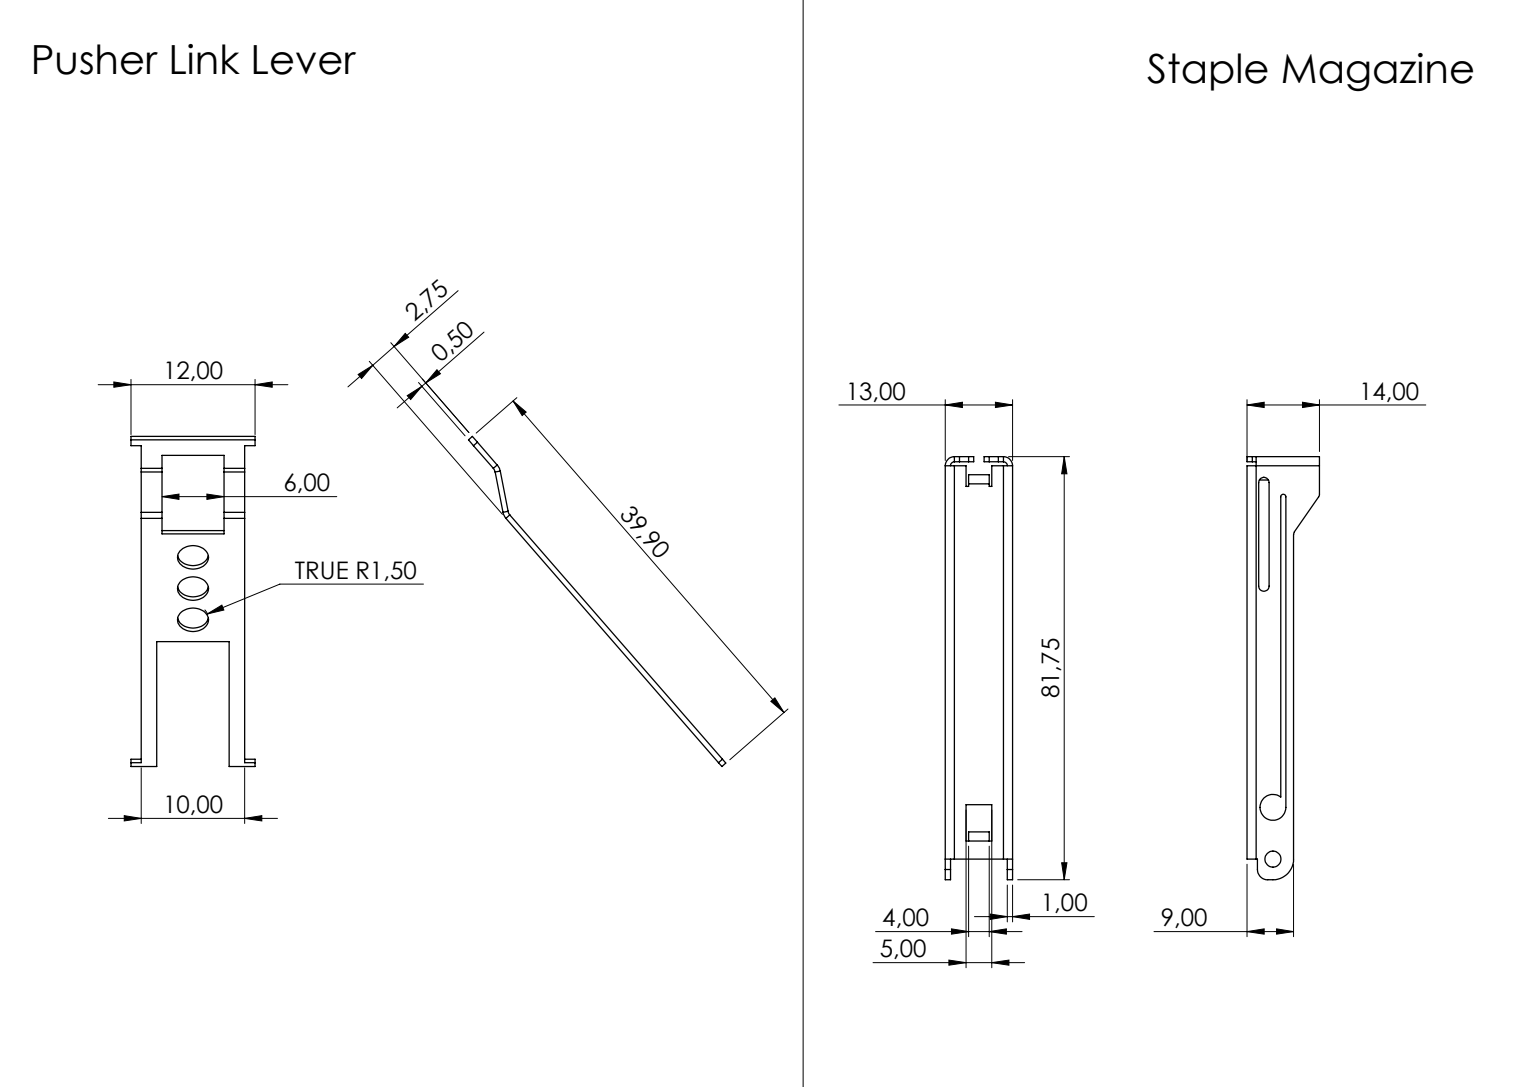
ISO-10303-21;
HEADER;
FILE_DESCRIPTION (('STEP AP214'),
    '1' );
FILE_NAME ('Pusher Link Lever.step',
    '2026-10-06T10:23:46',
    ( '' ),
    ( '' ),
    'SwSTEP 2.0',
    'SolidWorks 2020',
    '' );
FILE_SCHEMA (( 'AUTOMOTIVE_DESIGN' ));
ENDSEC;

DATA;
#10=VECTOR ( 'NONE', #20731, 1000.000000000000000 ) ;
#51=VECTOR ( 'NONE', #12391, 1000.000000000000227 ) ;
#60=CARTESIAN_POINT ( 'NONE',  ( 41.31606138205700063, 9.119667998728431257, 66.98393923633439329 ) ) ;
#67=CARTESIAN_POINT ( 'NONE',  ( 33.31606138205700773, -20.55619265724211076, 44.11584019928223910 ) ) ;
#85=CARTESIAN_POINT ( 'NONE',  ( 33.31606138205700773, -20.55619265724211076, 44.11584019928223910 ) ) ;
#88=CARTESIAN_POINT ( 'NONE',  ( 33.31606138205700773, 7.043113989679085307, 66.83274420321491505 ) ) ;
#111=EDGE_CURVE ( 'NONE', #24693, #6631, #6848, .T. ) ;
#114=EDGE_CURVE ( 'NONE', #23891, #14933, #22516, .T. ) ;
#137=SURFACE_STYLE_USAGE ( .BOTH. , #13306 ) ;
#149=DIRECTION ( 'NONE',  ( 0.000000000000000000, -0.7540134720837687876, -0.6568589528324780824 ) ) ;
#159=CARTESIAN_POINT ( 'NONE',  ( 41.31606138205700063, 7.187001342539796944, 66.09667597968754649 ) ) ;
#171=CARTESIAN_POINT ( 'NONE',  ( 43.31606138205700063, 3.536347952325769040, 64.10938348997790115 ) ) ;
#176=DIRECTION ( 'NONE',  ( 0.000000000000000000, 0.9814242980364923374, 0.1918498038142812112 ) ) ;
#215=LINE ( 'NONE', #15932, #731 ) ;
#239=ORIENTED_EDGE ( 'NONE', *, *, #12746, .F. ) ;
#276=CARTESIAN_POINT ( 'NONE',  ( 33.31606138205700773, -21.26162886970023536, 44.16441745890789150 ) ) ;
#333=EDGE_CURVE ( 'NONE', #14933, #7242, #7489, .T. ) ;
#339=EDGE_LOOP ( 'NONE', ( #14146, #23745, #1697, #21573 ) ) ;
#370=AXIS2_PLACEMENT_3D ( 'NONE', #22891, #22513, #18525 ) ;
#381=LINE ( 'NONE', #10079, #6023 ) ;
#388=ADVANCED_FACE ( 'NONE', ( #12254 ), #16230, .F. ) ;
#398=ORIENTED_EDGE ( 'NONE', *, *, #4868, .T. ) ;
#411=VECTOR ( 'NONE', #3457, 1000.000000000000227 ) ;
#416=DIRECTION ( 'NONE',  ( -1.000000000000000000, 0.000000000000000000, 0.000000000000000000 ) ) ;
#423=VECTOR ( 'NONE', #2307, 1000.000000000000000 ) ;
#432=EDGE_LOOP ( 'NONE', ( #18216, #5933, #5741, #16372 ) ) ;
#465=DIRECTION ( 'NONE',  ( 0.000000000000000000, -0.1918498038142812112, 0.9814242980364923374 ) ) ;
#484=DIRECTION ( 'NONE',  ( -1.000000000000000000, 0.000000000000000000, 0.000000000000000000 ) ) ;
#512=VECTOR ( 'NONE', #1905, 1000.000000000000227 ) ;
#522=DIRECTION ( 'NONE',  ( -1.000000000000000000, 0.000000000000000000, 0.000000000000000000 ) ) ;
#532=FACE_BOUND ( 'NONE', #6040, .T. ) ;
#572=CARTESIAN_POINT ( 'NONE',  ( 32.31606138205700063, -20.55619265724211076, 44.11584019928223910 ) ) ;
#583=EDGE_CURVE ( 'NONE', #22400, #7712, #22663, .T. ) ;
#586=DIRECTION ( 'NONE',  ( 0.000000000000000000, -0.7540134720837717852, -0.6568589528324746407 ) ) ;
#606=CARTESIAN_POINT ( 'NONE',  ( 41.31606138205700063, 7.864187680719676443, 65.89022736311019912 ) ) ;
#609=FACE_OUTER_BOUND ( 'NONE', #22404, .T. ) ;
#626=LINE ( 'NONE', #2187, #423 ) ;
#634=LINE ( 'NONE', #22037, #2547 ) ;
#649=EDGE_CURVE ( 'NONE', #18044, #10390, #12216, .T. ) ;
#676=DIRECTION ( 'NONE',  ( 1.000000000000000000, 0.000000000000000000, 0.000000000000000000 ) ) ;
#684=LINE ( 'NONE', #8319, #13350 ) ;
#692=EDGE_LOOP ( 'NONE', ( #13673, #1108, #11272, #13353 ) ) ;
#698=DIRECTION ( 'NONE',  ( 0.000000000000000000, -0.6568589528324746407, 0.7540134720837716742 ) ) ;
#708=PLANE ( 'NONE',  #13919 ) ;
#718=EDGE_LOOP ( 'NONE', ( #8864, #2817, #9327, #12481 ) ) ;
#731=VECTOR ( 'NONE', #465, 1000.000000000000227 ) ;
#746=ORIENTED_EDGE ( 'NONE', *, *, #3453, .F. ) ;
#758=EDGE_CURVE ( 'NONE', #12000, #4126, #215, .T. ) ;
#773=ORIENTED_EDGE ( 'NONE', *, *, #17559, .F. ) ;
#802=EDGE_CURVE ( 'NONE', #973, #13467, #6103, .T. ) ;
#815=ORIENTED_EDGE ( 'NONE', *, *, #8639, .F. ) ;
#866=ADVANCED_FACE ( 'NONE', ( #9118 ), #22748, .T. ) ;
#893=DIRECTION ( 'NONE',  ( -1.000000000000000000, 0.000000000000000000, 0.000000000000000000 ) ) ;
#909=CARTESIAN_POINT ( 'NONE',  ( 39.81606138205700063, -1.383222575549920119, 62.14461230196212682 ) ) ;
#963=CARTESIAN_POINT ( 'NONE',  ( 35.31606138205700773, 3.043703737701412226, 64.67489359404071081 ) ) ;
#970=CARTESIAN_POINT ( 'NONE',  ( 33.31606138205700773, 3.392460599465057403, 64.84545171350526971 ) ) ;
#973=VERTEX_POINT ( 'NONE', #15403 ) ;
#979=MECHANICAL_DESIGN_GEOMETRIC_PRESENTATION_REPRESENTATION('',(#16209),#14965);
#981=VERTEX_POINT ( 'NONE', #23370 ) ;
#995=FACE_BOUND ( 'NONE', #20971, .T. ) ;
#1028=ORIENTED_EDGE ( 'NONE', *, *, #24774, .T. ) ;
#1039=CARTESIAN_POINT ( 'NONE',  ( 41.31606138205700063, 8.104266321858618838, 55.82104096753806033 ) ) ;
#1091=CARTESIAN_POINT ( 'NONE',  ( 44.31606138205700063, 10.06218483883314718, 67.80501292737497465 ) ) ;
#1093=FACE_OUTER_BOUND ( 'NONE', #22758, .T. ) ;
#1095=DIRECTION ( 'NONE',  ( 0.000000000000000000, 0.7540134720837716742, 0.6568589528324746407 ) ) ;
#1108=ORIENTED_EDGE ( 'NONE', *, *, #23862, .T. ) ;
#1117=ADVANCED_FACE ( 'NONE', ( #22102 ), #16173, .F. ) ;
#1123=PLANE ( 'NONE',  #20476 ) ;
#1127=DIRECTION ( 'NONE',  ( 0.000000000000000000, 0.7540134720837716742, 0.6568589528324746407 ) ) ;
#1149=DIRECTION ( 'NONE',  ( 0.000000000000000000, 0.7540134720837716742, 0.6568589528324746407 ) ) ;
#1181=CIRCLE ( 'NONE', #15586, 1.500000000000001332 ) ;
#1206=FACE_OUTER_BOUND ( 'NONE', #18017, .T. ) ;
#1208=ORIENTED_EDGE ( 'NONE', *, *, #18160, .F. ) ;
#1241=ADVANCED_BREP_SHAPE_REPRESENTATION ( '', ( #17413, #2000 ), #7588 ) ;
#1245=ORIENTED_EDGE ( 'NONE', *, *, #19719, .F. ) ;
#1253=VECTOR ( 'NONE', #12245, 1000.000000000000227 ) ;
#1256=CARTESIAN_POINT ( 'NONE',  ( 33.31606138205700773, 10.62769494289597993, 68.29765714199933768 ) ) ;
#1260=LINE ( 'NONE', #24820, #4453 ) ;
#1265=CARTESIAN_POINT ( 'NONE',  ( 41.81606138205700063, -14.36460986495925241, 36.24727600202827915 ) ) ;
#1296=VERTEX_POINT ( 'NONE', #10772 ) ;
#1345=LINE ( 'NONE', #22733, #4452 ) ;
#1354=ORIENTED_EDGE ( 'NONE', *, *, #20276, .F. ) ;
#1382=ORIENTED_EDGE ( 'NONE', *, *, #10274, .T. ) ;
#1383=FACE_OUTER_BOUND ( 'NONE', #17604, .T. ) ;
#1395=EDGE_CURVE ( 'NONE', #20256, #6631, #1345, .T. ) ;
#1401=AXIS2_PLACEMENT_3D ( 'NONE', #3846, #7337, #9406 ) ;
#1404=ORIENTED_EDGE ( 'NONE', *, *, #22708, .F. ) ;
#1426=CARTESIAN_POINT ( 'NONE',  ( 43.31606138205700063, 7.535758204303438568, 66.26723409915207696 ) ) ;
#1453=ADVANCED_FACE ( 'NONE', ( #19133 ), #17457, .T. ) ;
#1471=FACE_OUTER_BOUND ( 'NONE', #24405, .T. ) ;
#1479=CARTESIAN_POINT ( 'NONE',  ( 33.31606138205700773, 7.282926244446933595, 65.60596383066929604 ) ) ;
#1497=CARTESIAN_POINT ( 'NONE',  ( 33.31606138205700773, -20.93319939328399926, 43.78741072286599945 ) ) ;
#1504=ADVANCED_FACE ( 'NONE', ( #3782 ), #23485, .F. ) ;
#1518=CARTESIAN_POINT ( 'NONE',  ( 33.31606138205700773, 7.535758204303438568, 66.26723409915207696 ) ) ;
#1524=CARTESIAN_POINT ( 'NONE',  ( 34.81606138205700773, -20.93319939328399926, 43.78741072286599945 ) ) ;
#1549=FACE_OUTER_BOUND ( 'NONE', #339, .T. ) ;
#1554=CARTESIAN_POINT ( 'NONE',  ( 33.31606138205700773, 7.864187680719676443, 65.89022736311019912 ) ) ;
#1555=EDGE_CURVE ( 'NONE', #18393, #21009, #3531, .T. ) ;
#1556=CARTESIAN_POINT ( 'NONE',  ( 35.31606138205700773, 7.283211578144648257, 66.04722806671131252 ) ) ;
#1567=CARTESIAN_POINT ( 'NONE',  ( 33.31606138205700773, 3.536347952325769040, 64.10938348997790115 ) ) ;
#1611=ORIENTED_EDGE ( 'NONE', *, *, #17429, .F. ) ;
#1641=FACE_OUTER_BOUND ( 'NONE', #23272, .T. ) ;
#1655=ORIENTED_EDGE ( 'NONE', *, *, #17523, .T. ) ;
#1664=EDGE_LOOP ( 'NONE', ( #7698, #19659, #15384, #19509 ) ) ;
#1697=ORIENTED_EDGE ( 'NONE', *, *, #18160, .T. ) ;
#1709=CARTESIAN_POINT ( 'NONE',  ( 38.31606138205700063, -4.399276463885007260, 59.51717649063222382 ) ) ;
#1710=VECTOR ( 'NONE', #11846, 1000.000000000000227 ) ;
#1719=ORIENTED_EDGE ( 'NONE', *, *, #7493, .T. ) ;
#1756=EDGE_CURVE ( 'NONE', #3936, #14994, #21690, .T. ) ;
#1793=VERTEX_POINT ( 'NONE', #4682 ) ;
#1808=VECTOR ( 'NONE', #12372, 1000.000000000000227 ) ;
#1812=CARTESIAN_POINT ( 'NONE',  ( 35.31606138205700773, 7.043113989679085307, 66.83274420321491505 ) ) ;
#1827=DIRECTION ( 'NONE',  ( 0.000000000000000000, 0.7540134720837716742, 0.6568589528324746407 ) ) ;
#1859=EDGE_CURVE ( 'NONE', #16267, #9779, #14977, .T. ) ;
#1867=ORIENTED_EDGE ( 'NONE', *, *, #17709, .T. ) ;
#1870=LINE ( 'NONE', #17869, #4225 ) ;
#1871=ORIENTED_EDGE ( 'NONE', *, *, #114, .T. ) ;
#1896=ORIENTED_EDGE ( 'NONE', *, *, #14372, .F. ) ;
#1905=DIRECTION ( 'NONE',  ( 5.421010862427517856E-17, -0.7540134720837717852, -0.6568589528324746407 ) ) ;
#1909=( LENGTH_UNIT ( ) NAMED_UNIT ( * ) SI_UNIT ( .MILLI., .METRE. ) );
#1912=DIRECTION ( 'NONE',  ( -1.000000000000000000, 0.000000000000000000, 0.000000000000000000 ) ) ;
#1916=DIRECTION ( 'NONE',  ( 0.000000000000000000, 0.7540134720837725624, 0.6568589528324736415 ) ) ;
#1919=ORIENTED_EDGE ( 'NONE', *, *, #12872, .F. ) ;
#1947=DIRECTION ( 'NONE',  ( 0.000000000000000000, 0.6568589528324746407, -0.7540134720837716742 ) ) ;
#1962=CARTESIAN_POINT ( 'NONE',  ( 35.31606138205700773, 8.104266321858618838, 55.82104096753806033 ) ) ;
#1979=EDGE_CURVE ( 'NONE', #2339, #23360, #5441, .T. ) ;
#1997=VERTEX_POINT ( 'NONE', #13310 ) ;
#2000=AXIS2_PLACEMENT_3D ( 'NONE', #9286, #12766, #22537 ) ;
#2004=DIRECTION ( 'NONE',  ( 1.000000000000000000, 0.000000000000000000, 0.000000000000000000 ) ) ;
#2032=VECTOR ( 'NONE', #13072, 1000.000000000000227 ) ;
#2046=AXIS2_PLACEMENT_3D ( 'NONE', #24848, #6964, #1149 ) ;
#2055=VECTOR ( 'NONE', #19199, 1000.000000000000227 ) ;
#2081=EDGE_CURVE ( 'NONE', #22220, #12980, #20869, .T. ) ;
#2084=EDGE_LOOP ( 'NONE', ( #8923, #5906, #22734, #17854 ) ) ;
#2088=PLANE ( 'NONE',  #25150 ) ;
#2111=EDGE_LOOP ( 'NONE', ( #21458, #24071, #20598, #8543 ) ) ;
#2116=ORIENTED_EDGE ( 'NONE', *, *, #7384, .F. ) ;
#2160=VECTOR ( 'NONE', #13117, 1000.000000000000000 ) ;
#2170=SURFACE_STYLE_USAGE ( .BOTH. , #11599 ) ;
#2178=VECTOR ( 'NONE', #12286, 1000.000000000000227 ) ;
#2187=CARTESIAN_POINT ( 'NONE',  ( 33.31606138205700773, 3.043703737701412226, 64.67489359404071081 ) ) ;
#2190=VERTEX_POINT ( 'NONE', #25289 ) ;
#2196=CARTESIAN_POINT ( 'NONE',  ( 38.31606138205700063, -1.054793099133682244, 61.76760556592023477 ) ) ;
#2222=ORIENTED_EDGE ( 'NONE', *, *, #20103, .F. ) ;
#2226=DIRECTION ( 'NONE',  ( 0.000000000000000000, 0.7540134720837717852, 0.6568589528324746407 ) ) ;
#2242=DIRECTION ( 'NONE',  ( 0.000000000000000000, -0.6568589528324746407, 0.7540134720837717852 ) ) ;
#2264=ORIENTED_EDGE ( 'NONE', *, *, #12872, .T. ) ;
#2265=CARTESIAN_POINT ( 'NONE',  ( 33.31606138205700773, 3.099306811489555891, 65.29760936252343129 ) ) ;
#2289=ADVANCED_FACE ( 'NONE', ( #15510 ), #13347, .T. ) ;
#2298=EDGE_LOOP ( 'NONE', ( #9215, #19456, #10247, #6097 ) ) ;
#2307=DIRECTION ( 'NONE',  ( 1.000000000000000000, 0.000000000000000000, 0.000000000000000000 ) ) ;
#2311=CARTESIAN_POINT ( 'NONE',  ( 43.31606138205700063, 2.715274261285174351, 65.05190033008260286 ) ) ;
#2339=VERTEX_POINT ( 'NONE', #4565 ) ;
#2366=CARTESIAN_POINT ( 'NONE',  ( 43.31606138205700063, 7.043113989679085307, 66.83274420321491505 ) ) ;
#2398=LINE ( 'NONE', #19807, #6565 ) ;
#2403=CARTESIAN_POINT ( 'NONE',  ( 44.31606138205700063, 10.62769494289597993, 68.29765714199933768 ) ) ;
#2409=DIRECTION ( 'NONE',  ( 0.000000000000000000, -0.6568589528324746407, 0.7540134720837717852 ) ) ;
#2420=CIRCLE ( 'NONE', #20143, 1.500000000000001332 ) ;
#2426=EDGE_LOOP ( 'NONE', ( #3479, #7297, #23375, #11174 ) ) ;
#2430=ORIENTED_EDGE ( 'NONE', *, *, #20190, .F. ) ;
#2440=CARTESIAN_POINT ( 'NONE',  ( 33.31606138205700773, -20.93319939328399926, 43.78741072286599945 ) ) ;
#2457=EDGE_CURVE ( 'NONE', #8692, #22403, #21950, .T. ) ;
#2488=ADVANCED_FACE ( 'NONE', ( #24748 ), #9075, .T. ) ;
#2511=ORIENTED_EDGE ( 'NONE', *, *, #19188, .T. ) ;
#2513=EDGE_LOOP ( 'NONE', ( #25331, #17268, #5891, #10881 ) ) ;
#2534=LINE ( 'NONE', #606, #24325 ) ;
#2547=VECTOR ( 'NONE', #4398, 1000.000000000000227 ) ;
#2554=CARTESIAN_POINT ( 'NONE',  ( 33.31606138205700773, 10.06218483883314718, 67.80501292737497465 ) ) ;
#2563=DIRECTION ( 'NONE',  ( 1.000000000000000000, 0.000000000000000000, 0.000000000000000000 ) ) ;
#2569=CARTESIAN_POINT ( 'NONE',  ( 41.31606138205700063, 7.282926244446937147, 65.60596383066929604 ) ) ;
#2572=VECTOR ( 'NONE', #586, 1000.000000000000227 ) ;
#2573=AXIS2_PLACEMENT_3D ( 'NONE', #16977, #2914, #7188 ) ;
#2591=PLANE ( 'NONE',  #21386 ) ;
#2592=CARTESIAN_POINT ( 'NONE',  ( 33.31606138205700773, 9.733755362416909307, 68.18201966341686671 ) ) ;
#2616=DIRECTION ( 'NONE',  ( 1.000000000000000000, 0.000000000000000000, 0.000000000000000000 ) ) ;
#2633=DIRECTION ( 'NONE',  ( 0.000000000000000000, -0.6568589528324746407, 0.7540134720837717852 ) ) ;
#2637=CARTESIAN_POINT ( 'NONE',  ( 34.81606138205700773, -14.36460986495925241, 36.24727600202827915 ) ) ;
#2639=DIRECTION ( 'NONE',  ( 1.000000000000000000, 0.000000000000000000, 0.000000000000000000 ) ) ;
#2667=ADVANCED_FACE ( 'NONE', ( #7502 ), #7762, .F. ) ;
#2677=CYLINDRICAL_SURFACE ( 'NONE', #16859, 1.500000000000001332 ) ;
#2679=ORIENTED_EDGE ( 'NONE', *, *, #22395, .T. ) ;
#2747=ORIENTED_EDGE ( 'NONE', *, *, #17523, .F. ) ;
#2785=EDGE_CURVE ( 'NONE', #14994, #22403, #21662, .T. ) ;
#2795=EDGE_CURVE ( 'NONE', #14933, #23891, #24552, .T. ) ;
#2797=EDGE_CURVE ( 'NONE', #24510, #23124, #12269, .T. ) ;
#2807=EDGE_LOOP ( 'NONE', ( #24648, #21947 ) ) ;
#2817=ORIENTED_EDGE ( 'NONE', *, *, #11715, .T. ) ;
#2825=LINE ( 'NONE', #18691, #10863 ) ;
#2892=PLANE ( 'NONE',  #9807 ) ;
#2897=LINE ( 'NONE', #8596, #20978 ) ;
#2914=DIRECTION ( 'NONE',  ( 1.000000000000000000, 0.000000000000000000, 0.000000000000000000 ) ) ;
#2937=DIRECTION ( 'NONE',  ( 0.000000000000000000, 0.7540134720837717852, 0.6568589528324745297 ) ) ;
#2965=ADVANCED_FACE ( 'NONE', ( #6079 ), #23962, .T. ) ;
#3009=VECTOR ( 'NONE', #8392, 1000.000000000000000 ) ;
#3043=VERTEX_POINT ( 'NONE', #14563 ) ;
#3061=ADVANCED_FACE ( 'NONE', ( #3088 ), #14685, .T. ) ;
#3064=CARTESIAN_POINT ( 'NONE',  ( 41.31606138205700063, 7.187001342539796944, 66.09667597968754649 ) ) ;
#3065=DIRECTION ( 'NONE',  ( 1.000000000000000000, 0.000000000000000000, 0.000000000000000000 ) ) ;
#3088=FACE_OUTER_BOUND ( 'NONE', #13458, .T. ) ;
#3150=CARTESIAN_POINT ( 'NONE',  ( 35.31606138205700773, 9.119667998728431257, 66.98393923633439329 ) ) ;
#3164=ORIENTED_EDGE ( 'NONE', *, *, #14530, .F. ) ;
#3174=ORIENTED_EDGE ( 'NONE', *, *, #22025, .F. ) ;
#3200=VECTOR ( 'NONE', #4429, 1000.000000000000227 ) ;
#3214=CARTESIAN_POINT ( 'NONE',  ( 35.31606138205700773, 7.282926244446937147, 65.60596383066929604 ) ) ;
#3233=PLANE ( 'NONE',  #23657 ) ;
#3245=DIRECTION ( 'NONE',  ( 0.000000000000000000, -0.7540134720837725624, -0.6568589528324736415 ) ) ;
#3291=CARTESIAN_POINT ( 'NONE',  ( 39.81606138205700063, -4.399276463885007260, 59.51717649063222382 ) ) ;
#3292=VECTOR ( 'NONE', #676, 1000.000000000000000 ) ;
#3304=ORIENTED_EDGE ( 'NONE', *, *, #20261, .T. ) ;
#3307=PLANE ( 'NONE',  #11587 ) ;
#3316=ADVANCED_FACE ( 'NONE', ( #21378 ), #13279, .F. ) ;
#3318=DIRECTION ( 'NONE',  ( 0.000000000000000000, 0.7540134720837716742, 0.6568589528324746407 ) ) ;
#3322=CARTESIAN_POINT ( 'NONE',  ( 38.31606138205700063, -7.415330352220093069, 56.88974067930232081 ) ) ;
#3353=EDGE_CURVE ( 'NONE', #17400, #19611, #1181, .T. ) ;
#3382=PRODUCT_CONTEXT ( 'NONE', #16546, 'mechanical' ) ;
#3389=DIRECTION ( 'NONE',  ( 0.000000000000000000, -0.7540134720837687876, -0.6568589528324780824 ) ) ;
#3403=ORIENTED_EDGE ( 'NONE', *, *, #14691, .F. ) ;
#3420=LINE ( 'NONE', #15017, #22147 ) ;
#3436=VECTOR ( 'NONE', #14093, 1000.000000000000227 ) ;
#3453=EDGE_CURVE ( 'NONE', #21357, #19154, #11862, .T. ) ;
#3454=DIRECTION ( 'NONE',  ( 0.000000000000000000, 0.6568589528324746407, -0.7540134720837717852 ) ) ;
#3457=DIRECTION ( 'NONE',  ( 0.000000000000000000, 0.7540134720837717852, 0.6568589528324746407 ) ) ;
#3479=ORIENTED_EDGE ( 'NONE', *, *, #17709, .F. ) ;
#3496=DIRECTION ( 'NONE',  ( 1.000000000000000000, 0.000000000000000000, 0.000000000000000000 ) ) ;
#3499=PRESENTATION_STYLE_ASSIGNMENT (( #137 ) ) ;
#3502=EDGE_CURVE ( 'NONE', #25135, #22767, #14035, .T. ) ;
#3517=ORIENTED_EDGE ( 'NONE', *, *, #24069, .F. ) ;
#3521=ORIENTED_EDGE ( 'NONE', *, *, #5510, .T. ) ;
#3523=DIRECTION ( 'NONE',  ( 0.000000000000000000, 0.7540134720837716742, 0.6568589528324746407 ) ) ;
#3531=LINE ( 'NONE', #11405, #13900 ) ;
#3564=DIRECTION ( 'NONE',  ( 0.000000000000000000, 0.1918498038142812112, -0.9814242980364923374 ) ) ;
#3586=AXIS2_PLACEMENT_3D ( 'NONE', #14833, #7241, #6984 ) ;
#3627=SHAPE_DEFINITION_REPRESENTATION ( #13836, #18165 ) ;
#3648=AXIS2_PLACEMENT_3D ( 'NONE', #15451, #11350, #17262 ) ;
#3657=DIRECTION ( 'NONE',  ( 0.000000000000000000, 0.6568589528324747517, -0.7540134720837717852 ) ) ;
#3663=ORIENTED_EDGE ( 'NONE', *, *, #11953, .T. ) ;
#3669=ORIENTED_EDGE ( 'NONE', *, *, #11478, .F. ) ;
#3677=CIRCLE ( 'NONE', #370, 0.7500000000000014433 ) ;
#3698=AXIS2_PLACEMENT_3D ( 'NONE', #2196, #17674, #4011 ) ;
#3707=CIRCLE ( 'NONE', #22642, 0.7500000000000014433 ) ;
#3716=CARTESIAN_POINT ( 'NONE',  ( 43.31606138205700063, 7.864187680719676443, 65.89022736311019912 ) ) ;
#3719=EDGE_CURVE ( 'NONE', #17105, #16154, #6279, .T. ) ;
#3721=FILL_AREA_STYLE ('',( #6179 ) ) ;
#3730=EDGE_CURVE ( 'NONE', #24147, #18393, #12212, .T. ) ;
#3782=FACE_OUTER_BOUND ( 'NONE', #23471, .T. ) ;
#3793=CARTESIAN_POINT ( 'NONE',  ( 33.31606138205700773, 7.187001342539796944, 66.09667597968754649 ) ) ;
#3797=CARTESIAN_POINT ( 'NONE',  ( 41.31606138205700063, 3.392460599465057403, 64.84545171350526971 ) ) ;
#3801=CARTESIAN_POINT ( 'NONE',  ( 41.31606138205700063, 7.283211578144648257, 66.04722806671131252 ) ) ;
#3811=PLANE ( 'NONE',  #7511 ) ;
#3844=ORIENTED_EDGE ( 'NONE', *, *, #9003, .F. ) ;
#3846=CARTESIAN_POINT ( 'NONE',  ( 41.31606138205700063, 8.104266321858618838, 55.82104096753806033 ) ) ;
#3850=CARTESIAN_POINT ( 'NONE',  ( 33.31606138205700773, -20.88462213365835041, 44.49284693532412405 ) ) ;
#3907=EDGE_CURVE ( 'NONE', #10892, #20855, #23427, .T. ) ;
#3921=VECTOR ( 'NONE', #4641, 1000.000000000000000 ) ;
#3936=VERTEX_POINT ( 'NONE', #5789 ) ;
#3946=FACE_OUTER_BOUND ( 'NONE', #19029, .T. ) ;
#4011=DIRECTION ( 'NONE',  ( -1.000000000000000000, 0.000000000000000000, 0.000000000000000000 ) ) ;
#4012=CARTESIAN_POINT ( 'NONE',  ( 39.81606138205700063, -1.054793099133682244, 61.76760556592023477 ) ) ;
#4016=CARTESIAN_POINT ( 'NONE',  ( 33.31606138205700773, -21.26162886970023536, 44.16441745890789150 ) ) ;
#4042=CARTESIAN_POINT ( 'NONE',  ( 41.81606138205700063, -14.36460986495925241, 36.24727600202827915 ) ) ;
#4057=CARTESIAN_POINT ( 'NONE',  ( 43.31606138205700063, 3.043703737701412226, 64.67489359404071081 ) ) ;
#4064=DIRECTION ( 'NONE',  ( 0.000000000000000000, 0.6568589528324745297, -0.7540134720837717852 ) ) ;
#4065=ORIENTED_EDGE ( 'NONE', *, *, #24069, .T. ) ;
#4095=CARTESIAN_POINT ( 'NONE',  ( 35.31606138205700773, 3.392460599465057403, 64.84545171350526971 ) ) ;
#4110=AXIS2_PLACEMENT_3D ( 'NONE', #11177, #21088, #7042 ) ;
#4114=EDGE_CURVE ( 'NONE', #6859, #24693, #15194, .T. ) ;
#4119=CIRCLE ( 'NONE', #3698, 1.500000000000001332 ) ;
#4120=DIRECTION ( 'NONE',  ( 0.000000000000000000, 0.6568589528324746407, -0.7540134720837716742 ) ) ;
#4126=VERTEX_POINT ( 'NONE', #19027 ) ;
#4152=DIRECTION ( 'NONE',  ( 0.000000000000000000, -0.6568589528324746407, 0.7540134720837716742 ) ) ;
#4159=DIRECTION ( 'NONE',  ( 0.000000000000000000, 0.7540134720837717852, 0.6568589528324745297 ) ) ;
#4170=ORIENTED_EDGE ( 'NONE', *, *, #10595, .F. ) ;
#4181=CARTESIAN_POINT ( 'NONE',  ( 44.31606138205700063, -20.93319939328399926, 43.78741072286599945 ) ) ;
#4188=LINE ( 'NONE', #4057, #10491 ) ;
#4217=CARTESIAN_POINT ( 'NONE',  ( 39.81606138205700063, -7.415330352220093069, 56.88974067930232081 ) ) ;
#4225=VECTOR ( 'NONE', #11817, 1000.000000000000000 ) ;
#4232=EDGE_CURVE ( 'NONE', #10390, #2339, #4704, .T. ) ;
#4233=EDGE_LOOP ( 'NONE', ( #10281, #1028, #23778, #3174 ) ) ;
#4245=CARTESIAN_POINT ( 'NONE',  ( 41.81606138205700063, -9.197413316359888569, 54.67416070422748220 ) ) ;
#4279=CARTESIAN_POINT ( 'NONE',  ( 33.31606138205700773, 3.099306811489555891, 65.29760936252343129 ) ) ;
#4298=VECTOR ( 'NONE', #6505, 1000.000000000000227 ) ;
#4348=CARTESIAN_POINT ( 'NONE',  ( 33.31606138205700773, -8.868983839943650693, 54.29715396818559725 ) ) ;
#4369=EDGE_CURVE ( 'NONE', #23360, #22220, #7265, .T. ) ;
#4383=VERTEX_POINT ( 'NONE', #10883 ) ;
#4398=DIRECTION ( 'NONE',  ( 0.000000000000000000, -0.7540134720837717852, -0.6568589528324746407 ) ) ;
#4422=ORIENTED_EDGE ( 'NONE', *, *, #14978, .T. ) ;
#4429=DIRECTION ( 'NONE',  ( 0.000000000000000000, -0.6568589528324746407, 0.7540134720837717852 ) ) ;
#4452=VECTOR ( 'NONE', #5098, 1000.000000000000227 ) ;
#4453=VECTOR ( 'NONE', #10201, 1000.000000000000227 ) ;
#4455=ORIENTED_EDGE ( 'NONE', *, *, #19188, .F. ) ;
#4477=DIRECTION ( 'NONE',  ( 0.000000000000000000, 0.7540134720837717852, 0.6568589528324746407 ) ) ;
#4488=ORIENTED_EDGE ( 'NONE', *, *, #10233, .T. ) ;
#4503=ORIENTED_EDGE ( 'NONE', *, *, #333, .F. ) ;
#4515=DIRECTION ( 'NONE',  ( 0.000000000000000000, 0.7540134720837717852, 0.6568589528324747517 ) ) ;
#4522=EDGE_CURVE ( 'NONE', #22473, #18865, #7907, .T. ) ;
#4545=EDGE_LOOP ( 'NONE', ( #11039, #7124, #17534, #14179 ) ) ;
#4565=CARTESIAN_POINT ( 'NONE',  ( 35.31606138205700773, 8.791238522312193382, 67.36094597237627113 ) ) ;
#4587=CARTESIAN_POINT ( 'NONE',  ( 41.31606138205700063, 8.104266321858618838, 55.82104096753806033 ) ) ;
#4641=DIRECTION ( 'NONE',  ( 0.000000000000000000, 0.6568589528324745297, -0.7540134720837717852 ) ) ;
#4682=CARTESIAN_POINT ( 'NONE',  ( 43.31606138205700063, 3.043703737701412226, 64.67489359404071081 ) ) ;
#4686=VECTOR ( 'NONE', #23429, 1000.000000000000227 ) ;
#4692=ADVANCED_FACE ( 'NONE', ( #8540 ), #2591, .T. ) ;
#4695=EDGE_CURVE ( 'NONE', #1997, #21009, #18451, .T. ) ;
#4697=EDGE_CURVE ( 'NONE', #10390, #22220, #6597, .T. ) ;
#4704=LINE ( 'NONE', #24008, #11115 ) ;
#4710=PLANE ( 'NONE',  #5794 ) ;
#4711=DIRECTION ( 'NONE',  ( 0.000000000000000000, -0.6568589528324746407, 0.7540134720837717852 ) ) ;
#4721=ORIENTED_EDGE ( 'NONE', *, *, #19719, .T. ) ;
#4726=DIRECTION ( 'NONE',  ( 0.000000000000000000, 0.7540134720837716742, 0.6568589528324746407 ) ) ;
#4761=CARTESIAN_POINT ( 'NONE',  ( 33.31606138205700773, 7.187001342539796944, 66.09667597968754649 ) ) ;
#4767=DIRECTION ( 'NONE',  ( 0.000000000000000000, 0.6568589528324746407, -0.7540134720837717852 ) ) ;
#4790=ORIENTED_EDGE ( 'NONE', *, *, #10497, .F. ) ;
#4807=AXIS2_PLACEMENT_3D ( 'NONE', #1567, #11132, #3389 ) ;
#4834=ORIENTED_EDGE ( 'NONE', *, *, #10977, .F. ) ;
#4835=ORIENTED_EDGE ( 'NONE', *, *, #11953, .F. ) ;
#4844=ADVANCED_FACE ( 'NONE', ( #15085 ), #8673, .T. ) ;
#4854=CARTESIAN_POINT ( 'NONE',  ( 33.31606138205700773, 7.043113989679085307, 66.83274420321491505 ) ) ;
#4868=EDGE_CURVE ( 'NONE', #17400, #973, #16503, .T. ) ;
#4869=VECTOR ( 'NONE', #5487, 1000.000000000000227 ) ;
#4875=AXIS2_PLACEMENT_3D ( 'NONE', #1962, #6447, #8510 ) ;
#4876=CYLINDRICAL_SURFACE ( 'NONE', #9436, 1.500000000000001332 ) ;
#4895=CARTESIAN_POINT ( 'NONE',  ( 41.31606138205700063, 2.715274261285174351, 65.05190033008260286 ) ) ;
#4900=CIRCLE ( 'NONE', #12740, 0.7500000000000041078 ) ;
#4921=VECTOR ( 'NONE', #11743, 1000.000000000000227 ) ;
#4923=EDGE_LOOP ( 'NONE', ( #17633, #2511, #1354, #7095 ) ) ;
#4937=DIRECTION ( 'NONE',  ( 1.000000000000000000, 0.000000000000000000, 0.000000000000000000 ) ) ;
#4967=ORIENTED_EDGE ( 'NONE', *, *, #12217, .F. ) ;
#4969=VECTOR ( 'NONE', #7568, 1000.000000000000227 ) ;
#4976=FACE_OUTER_BOUND ( 'NONE', #24006, .T. ) ;
#4990=LINE ( 'NONE', #16709, #23954 ) ;
#4996=CARTESIAN_POINT ( 'NONE',  ( 38.31606138205700063, -1.383222575549920119, 62.14461230196212682 ) ) ;
#5048=DIRECTION ( 'NONE',  ( 1.000000000000000000, 0.000000000000000000, 0.000000000000000000 ) ) ;
#5060=AXIS2_PLACEMENT_3D ( 'NONE', #8855, #14763, #5231 ) ;
#5062=VECTOR ( 'NONE', #25157, 1000.000000000000227 ) ;
#5096=CARTESIAN_POINT ( 'NONE',  ( 35.31606138205700773, 8.104266321858618838, 55.82104096753806033 ) ) ;
#5098=DIRECTION ( 'NONE',  ( 0.000000000000000000, 0.1918498038142812112, -0.9814242980364923374 ) ) ;
#5112=DIRECTION ( 'NONE',  ( -1.000000000000000000, 0.000000000000000000, 0.000000000000000000 ) ) ;
#5141=CARTESIAN_POINT ( 'NONE',  ( 41.31606138205700063, 8.104266321858618838, 55.82104096753806033 ) ) ;
#5145=PLANE ( 'NONE',  #21410 ) ;
#5152=ORIENTED_EDGE ( 'NONE', *, *, #14691, .T. ) ;
#5173=CARTESIAN_POINT ( 'NONE',  ( 41.81606138205700063, -9.197413316359888569, 54.67416070422748220 ) ) ;
#5186=ORIENTED_EDGE ( 'NONE', *, *, #7384, .T. ) ;
#5230=CARTESIAN_POINT ( 'NONE',  ( 44.31606138205700063, 9.733755362416909307, 68.18201966341686671 ) ) ;
#5231=DIRECTION ( 'NONE',  ( -1.000000000000000000, 0.000000000000000000, 0.000000000000000000 ) ) ;
#5233=DIRECTION ( 'NONE',  ( 0.000000000000000000, 0.6568589528324747517, -0.7540134720837718962 ) ) ;
#5251=CARTESIAN_POINT ( 'NONE',  ( 33.31606138205700773, 7.535758204303438568, 66.26723409915207696 ) ) ;
#5289=ORIENTED_EDGE ( 'NONE', *, *, #23265, .T. ) ;
#5297=DIRECTION ( 'NONE',  ( 1.000000000000000000, 0.000000000000000000, 0.000000000000000000 ) ) ;
#5298=EDGE_CURVE ( 'NONE', #19154, #22473, #626, .T. ) ;
#5319=CARTESIAN_POINT ( 'NONE',  ( 35.31606138205700773, 7.043113989679085307, 66.83274420321491505 ) ) ;
#5320=VECTOR ( 'NONE', #19804, 1000.000000000000227 ) ;
#5329=CARTESIAN_POINT ( 'NONE',  ( 43.31606138205700063, 10.06218483883314718, 67.80501292737497465 ) ) ;
#5346=ORIENTED_EDGE ( 'NONE', *, *, #2785, .F. ) ;
#5354=CARTESIAN_POINT ( 'NONE',  ( 35.31606138205700773, 3.296535697557906985, 65.33616386252352015 ) ) ;
#5362=DIRECTION ( 'NONE',  ( 1.000000000000000000, 0.000000000000000000, 0.000000000000000000 ) ) ;
#5367=VERTEX_POINT ( 'NONE', #16868 ) ;
#5384=ADVANCED_FACE ( 'NONE', ( #10701 ), #20607, .T. ) ;
#5388=DIRECTION ( 'NONE',  ( -0.000000000000000000, -0.9814242980364923374, -0.1918498038142812112 ) ) ;
#5393=CARTESIAN_POINT ( 'NONE',  ( 36.81606138205700063, -7.415330352220093069, 56.88974067930232081 ) ) ;
#5420=CARTESIAN_POINT ( 'NONE',  ( 36.81606138205700063, -1.383222575549920119, 62.14461230196212682 ) ) ;
#5441=LINE ( 'NONE', #1556, #18388 ) ;
#5464=DIRECTION ( 'NONE',  ( 0.000000000000000000, 0.6568589528324747517, -0.7540134720837717852 ) ) ;
#5487=DIRECTION ( 'NONE',  ( -5.421010862427517856E-17, 0.7540134720837717852, 0.6568589528324746407 ) ) ;
#5499=DIRECTION ( 'NONE',  ( 0.000000000000000000, -0.7540134720837717852, -0.6568589528324746407 ) ) ;
#5504=EDGE_LOOP ( 'NONE', ( #7618, #9747, #20329, #5152 ) ) ;
#5510=EDGE_CURVE ( 'NONE', #9479, #9779, #17000, .T. ) ;
#5569=CARTESIAN_POINT ( 'NONE',  ( 43.31606138205700063, 9.733755362416909307, 68.18201966341686671 ) ) ;
#5580=CARTESIAN_POINT ( 'NONE',  ( 38.31606138205700063, -3.742417511052531509, 58.76316301854844681 ) ) ;
#5582=CYLINDRICAL_SURFACE ( 'NONE', #4807, 0.7500000000000027756 ) ;
#5598=CARTESIAN_POINT ( 'NONE',  ( 33.31606138205700773, 7.043113989679085307, 66.83274420321491505 ) ) ;
#5605=DIRECTION ( 'NONE',  ( 1.000000000000000000, 0.000000000000000000, 0.000000000000000000 ) ) ;
#5606=LINE ( 'NONE', #21319, #4869 ) ;
#5639=CIRCLE ( 'NONE', #6869, 1.500000000000001332 ) ;
#5645=CARTESIAN_POINT ( 'NONE',  ( 38.31606138205700063, -7.086900875803856970, 56.51273394326043586 ) ) ;
#5655=AXIS2_PLACEMENT_3D ( 'NONE', #21412, #11634, #14197 ) ;
#5666=CARTESIAN_POINT ( 'NONE',  ( 33.31606138205700773, 3.536347952325769040, 64.10938348997790115 ) ) ;
#5701=LINE ( 'NONE', #11516, #12718 ) ;
#5703=CIRCLE ( 'NONE', #20105, 1.249999999999996891 ) ;
#5740=DIRECTION ( 'NONE',  ( 1.000000000000000000, 0.000000000000000000, 0.000000000000000000 ) ) ;
#5741=ORIENTED_EDGE ( 'NONE', *, *, #12746, .T. ) ;
#5764=LINE ( 'NONE', #21346, #19430 ) ;
#5766=ADVANCED_FACE ( 'NONE', ( #8840 ), #4710, .F. ) ;
#5773=DIRECTION ( 'NONE',  ( 0.000000000000000000, -0.6568589528324746407, 0.7540134720837717852 ) ) ;
#5783=ORIENTED_EDGE ( 'NONE', *, *, #583, .F. ) ;
#5788=DIRECTION ( 'NONE',  ( 0.000000000000000000, -0.6568589528324746407, 0.7540134720837717852 ) ) ;
#5789=CARTESIAN_POINT ( 'NONE',  ( 41.81606138205700063, -20.93319939328399926, 43.78741072286599945 ) ) ;
#5790=CARTESIAN_POINT ( 'NONE',  ( 41.31606138205700063, 8.791238522312193382, 67.36094597237627113 ) ) ;
#5791=PLANE ( 'NONE',  #19087 ) ;
#5794=AXIS2_PLACEMENT_3D ( 'NONE', #23893, #6257, #24134 ) ;
#5847=CARTESIAN_POINT ( 'NONE',  ( 33.31606138205700773, 7.043113989679085307, 66.83274420321491505 ) ) ;
#5849=EDGE_CURVE ( 'NONE', #17790, #13140, #14247, .T. ) ;
#5855=DIRECTION ( 'NONE',  ( -1.000000000000000000, 0.000000000000000000, 0.000000000000000000 ) ) ;
#5891=ORIENTED_EDGE ( 'NONE', *, *, #22166, .F. ) ;
#5896=VECTOR ( 'NONE', #19766, 1000.000000000000000 ) ;
#5906=ORIENTED_EDGE ( 'NONE', *, *, #2081, .T. ) ;
#5930=DIRECTION ( 'NONE',  ( -1.000000000000000000, 0.000000000000000000, 0.000000000000000000 ) ) ;
#5933=ORIENTED_EDGE ( 'NONE', *, *, #14978, .F. ) ;
#5934=VERTEX_POINT ( 'NONE', #12954 ) ;
#5946=PLANE ( 'NONE',  #14547 ) ;
#5960=ADVANCED_FACE ( 'NONE', ( #1206 ), #23102, .F. ) ;
#5986=ORIENTED_EDGE ( 'NONE', *, *, #2797, .F. ) ;
#5987=DIRECTION ( 'NONE',  ( 0.000000000000000000, -0.7540134720837697868, -0.6568589528324768612 ) ) ;
#6019=LINE ( 'NONE', #6521, #18250 ) ;
#6023=VECTOR ( 'NONE', #14060, 1000.000000000000000 ) ;
#6040=EDGE_LOOP ( 'NONE', ( #6384, #1871 ) ) ;
#6044=CARTESIAN_POINT ( 'NONE',  ( 44.31606138205700063, 10.06218483883314718, 67.80501292737497465 ) ) ;
#6047=FACE_OUTER_BOUND ( 'NONE', #5504, .T. ) ;
#6048=( LENGTH_UNIT ( ) NAMED_UNIT ( * ) SI_UNIT ( .MILLI., .METRE. ) );
#6049=AXIS2_PLACEMENT_3D ( 'NONE', #21576, #3657, #21196 ) ;
#6071=CARTESIAN_POINT ( 'NONE',  ( 44.31606138205700063, 10.06218483883314718, 67.80501292737497465 ) ) ;
#6072=EDGE_CURVE ( 'NONE', #12980, #5934, #23617, .T. ) ;
#6079=FACE_OUTER_BOUND ( 'NONE', #8197, .T. ) ;
#6081=VECTOR ( 'NONE', #10403, 1000.000000000000000 ) ;
#6094=ORIENTED_EDGE ( 'NONE', *, *, #9587, .T. ) ;
#6095=DIRECTION ( 'NONE',  ( 0.000000000000000000, 0.7540134720837716742, 0.6568589528324746407 ) ) ;
#6097=ORIENTED_EDGE ( 'NONE', *, *, #583, .T. ) ;
#6103=CIRCLE ( 'NONE', #15961, 1.500000000000001332 ) ;
#6145=VERTEX_POINT ( 'NONE', #15376 ) ;
#6163=ORIENTED_EDGE ( 'NONE', *, *, #23820, .F. ) ;
#6177=CIRCLE ( 'NONE', #11105, 1.249999999999998890 ) ;
#6179=FILL_AREA_STYLE_COLOUR ( '', #21977 ) ;
#6182=DIRECTION ( 'NONE',  ( 0.000000000000000000, 0.6568589528324747517, -0.7540134720837718962 ) ) ;
#6208=CARTESIAN_POINT ( 'NONE',  ( 35.31606138205700773, 8.104266321858618838, 55.82104096753806033 ) ) ;
#6216=CARTESIAN_POINT ( 'NONE',  ( 44.31606138205700063, -21.26162886970023536, 44.16441745890789150 ) ) ;
#6217=VECTOR ( 'NONE', #2633, 1000.000000000000227 ) ;
#6223=FACE_OUTER_BOUND ( 'NONE', #24949, .T. ) ;
#6227=ORIENTED_EDGE ( 'NONE', *, *, #18105, .F. ) ;
#6236=ORIENTED_EDGE ( 'NONE', *, *, #24117, .F. ) ;
#6237=CARTESIAN_POINT ( 'NONE',  ( 33.31606138205700773, 7.283211578144648257, 66.04722806671131252 ) ) ;
#6241=ORIENTED_EDGE ( 'NONE', *, *, #7493, .F. ) ;
#6257=DIRECTION ( 'NONE',  ( 0.000000000000000000, 0.1918498038142811835, -0.9814242980364923374 ) ) ;
#6259=ORIENTED_EDGE ( 'NONE', *, *, #649, .F. ) ;
#6279=LINE ( 'NONE', #13881, #5320 ) ;
#6284=DIRECTION ( 'NONE',  ( 0.000000000000000000, -0.6568589528324746407, 0.7540134720837717852 ) ) ;
#6290=DIRECTION ( 'NONE',  ( 0.000000000000000000, 0.6568589528324746407, -0.7540134720837717852 ) ) ;
#6292=ORIENTED_EDGE ( 'NONE', *, *, #24317, .T. ) ;
#6303=DIRECTION ( 'NONE',  ( -1.000000000000000000, 0.000000000000000000, 0.000000000000000000 ) ) ;
#6330=CARTESIAN_POINT ( 'NONE',  ( 43.31606138205700063, 3.536347952325769040, 64.10938348997790115 ) ) ;
#6358=PLANE ( 'NONE',  #8362 ) ;
#6384=ORIENTED_EDGE ( 'NONE', *, *, #2795, .T. ) ;
#6398=DIRECTION ( 'NONE',  ( 1.000000000000000000, 4.087515222582816494E-17, 3.560839518387611236E-17 ) ) ;
#6399=ADVANCED_FACE ( 'NONE', ( #24866 ), #3233, .T. ) ;
#6404=PLANE ( 'NONE',  #7545 ) ;
#6447=DIRECTION ( 'NONE',  ( 1.000000000000000000, 0.000000000000000000, 0.000000000000000000 ) ) ;
#6470=ORIENTED_EDGE ( 'NONE', *, *, #8946, .T. ) ;
#6474=FACE_OUTER_BOUND ( 'NONE', #24445, .T. ) ;
#6489=AXIS2_PLACEMENT_3D ( 'NONE', #1497, #11192, #3318 ) ;
#6495=LINE ( 'NONE', #6751, #2055 ) ;
#6500=CARTESIAN_POINT ( 'NONE',  ( 32.31606138205700063, -20.55619265724211076, 44.11584019928223910 ) ) ;
#6505=DIRECTION ( 'NONE',  ( 0.000000000000000000, -0.7540134720837717852, -0.6568589528324746407 ) ) ;
#6515=APPLICATION_CONTEXT ( 'automotive_design' ) ;
#6521=CARTESIAN_POINT ( 'NONE',  ( 41.31606138205700063, 1.207247317117632335, 63.73818242441765847 ) ) ;
#6539=ORIENTED_EDGE ( 'NONE', *, *, #24117, .T. ) ;
#6551=VECTOR ( 'NONE', #8113, 1000.000000000000000 ) ;
#6565=VECTOR ( 'NONE', #6284, 1000.000000000000227 ) ;
#6597=LINE ( 'NONE', #21807, #24659 ) ;
#6631=VERTEX_POINT ( 'NONE', #17286 ) ;
#6662=ORIENTED_EDGE ( 'NONE', *, *, #111, .T. ) ;
#6681=CARTESIAN_POINT ( 'NONE',  ( 33.31606138205700773, 3.392460599465057403, 64.84545171350526971 ) ) ;
#6744=CARTESIAN_POINT ( 'NONE',  ( 41.81606138205700063, -8.868983839943650693, 54.29715396818559725 ) ) ;
#6749=CYLINDRICAL_SURFACE ( 'NONE', #9422, 1.249999999999998668 ) ;
#6751=CARTESIAN_POINT ( 'NONE',  ( 33.31606138205700773, -20.93319939328399926, 43.78741072286599945 ) ) ;
#6762=EDGE_CURVE ( 'NONE', #14130, #22400, #20357, .T. ) ;
#6767=CARTESIAN_POINT ( 'NONE',  ( 33.31606138205700773, 7.864187680719676443, 65.89022736311019912 ) ) ;
#6848=LINE ( 'NONE', #20774, #9788 ) ;
#6859=VERTEX_POINT ( 'NONE', #9288 ) ;
#6864=AXIS2_PLACEMENT_3D ( 'NONE', #18369, #2639, #22229 ) ;
#6869=AXIS2_PLACEMENT_3D ( 'NONE', #10755, #6873, #8947 ) ;
#6873=DIRECTION ( 'NONE',  ( 0.000000000000000000, 0.6568589528324747517, -0.7540134720837718962 ) ) ;
#6884=ORIENTED_EDGE ( 'NONE', *, *, #11715, .F. ) ;
#6886=DIRECTION ( 'NONE',  ( -1.000000000000000000, 0.000000000000000000, 0.000000000000000000 ) ) ;
#6902=DIRECTION ( 'NONE',  ( -1.000000000000000000, 0.000000000000000000, 0.000000000000000000 ) ) ;
#6914=ADVANCED_FACE ( 'NONE', ( #18551 ), #24836, .T. ) ;
#6918=PLANE ( 'NONE',  #17782 ) ;
#6922=ORIENTED_EDGE ( 'NONE', *, *, #4697, .T. ) ;
#6951=CARTESIAN_POINT ( 'NONE',  ( 44.31606138205700063, -20.55619265724211076, 44.11584019928223910 ) ) ;
#6958=AXIS2_PLACEMENT_3D ( 'NONE', #21015, #5297, #15080 ) ;
#6964=DIRECTION ( 'NONE',  ( -1.000000000000000000, 0.000000000000000000, 0.000000000000000000 ) ) ;
#6975=VECTOR ( 'NONE', #16454, 1000.000000000000000 ) ;
#6984=DIRECTION ( 'NONE',  ( -1.000000000000000000, 0.000000000000000000, 0.000000000000000000 ) ) ;
#7032=CIRCLE ( 'NONE', #10325, 1.249999999999996891 ) ;
#7042=DIRECTION ( 'NONE',  ( 0.000000000000000000, 0.7540134720837687876, 0.6568589528324780824 ) ) ;
#7065=FACE_OUTER_BOUND ( 'NONE', #17101, .T. ) ;
#7077=EDGE_LOOP ( 'NONE', ( #4422, #23654, #11079, #12328 ) ) ;
#7088=VECTOR ( 'NONE', #12482, 1000.000000000000227 ) ;
#7095=ORIENTED_EDGE ( 'NONE', *, *, #20949, .T. ) ;
#7112=CIRCLE ( 'NONE', #9169, 1.249999999999998668 ) ;
#7124=ORIENTED_EDGE ( 'NONE', *, *, #7926, .F. ) ;
#7157=EDGE_LOOP ( 'NONE', ( #773, #23363, #4834, #11420 ) ) ;
#7187=AXIS2_PLACEMENT_3D ( 'NONE', #17072, #5464, #3523 ) ;
#7188=DIRECTION ( 'NONE',  ( 0.000000000000000000, 0.7540134720837717852, 0.6568589528324747517 ) ) ;
#7194=PLANE ( 'NONE',  #6489 ) ;
#7201=CARTESIAN_POINT ( 'NONE',  ( 33.31606138205700773, 7.864187680719676443, 65.89022736311019912 ) ) ;
#7214=DIRECTION ( 'NONE',  ( 0.000000000000000000, 0.7540134720837716742, 0.6568589528324746407 ) ) ;
#7229=EDGE_LOOP ( 'NONE', ( #23479, #22342, #6662, #4170 ) ) ;
#7241=DIRECTION ( 'NONE',  ( 0.000000000000000000, 0.6568589528324747517, -0.7540134720837718962 ) ) ;
#7242=VERTEX_POINT ( 'NONE', #12491 ) ;
#7243=DIRECTION ( 'NONE',  ( -1.000000000000000000, 0.000000000000000000, 0.000000000000000000 ) ) ;
#7265=LINE ( 'NONE', #24505, #2032 ) ;
#7277=PLANE ( 'NONE',  #11302 ) ;
#7278=ADVANCED_FACE ( 'NONE', ( #609 ), #21883, .T. ) ;
#7287=ORIENTED_EDGE ( 'NONE', *, *, #8946, .F. ) ;
#7297=ORIENTED_EDGE ( 'NONE', *, *, #10977, .T. ) ;
#7326=LINE ( 'NONE', #18924, #10 ) ;
#7337=DIRECTION ( 'NONE',  ( 0.000000000000000000, 0.7540134720837717852, 0.6568589528324747517 ) ) ;
#7384=EDGE_CURVE ( 'NONE', #8218, #7685, #11651, .T. ) ;
#7397=ORIENTED_EDGE ( 'NONE', *, *, #9353, .F. ) ;
#7441=VECTOR ( 'NONE', #20087, 1000.000000000000000 ) ;
#7467=ORIENTED_EDGE ( 'NONE', *, *, #19005, .F. ) ;
#7470=FACE_OUTER_BOUND ( 'NONE', #7157, .T. ) ;
#7489=LINE ( 'NONE', #10313, #15948 ) ;
#7493=EDGE_CURVE ( 'NONE', #16518, #23360, #24428, .T. ) ;
#7502=FACE_OUTER_BOUND ( 'NONE', #692, .T. ) ;
#7510=DIRECTION ( 'NONE',  ( -1.000000000000000000, 0.000000000000000000, 0.000000000000000000 ) ) ;
#7511=AXIS2_PLACEMENT_3D ( 'NONE', #19787, #19534, #11696 ) ;
#7534=AXIS2_PLACEMENT_3D ( 'NONE', #8550, #2004, #12426 ) ;
#7537=VECTOR ( 'NONE', #176, 1000.000000000000227 ) ;
#7538=CARTESIAN_POINT ( 'NONE',  ( 39.81606138205700063, -7.086900875803856970, 56.51273394326043586 ) ) ;
#7543=LINE ( 'NONE', #15134, #19897 ) ;
#7545=AXIS2_PLACEMENT_3D ( 'NONE', #2265, #10141, #14133 ) ;
#7568=DIRECTION ( 'NONE',  ( 0.000000000000000000, 0.7540134720837717852, 0.6568589528324746407 ) ) ;
#7580=EDGE_CURVE ( 'NONE', #18044, #9433, #25053, .T. ) ;
#7582=FACE_BOUND ( 'NONE', #15241, .T. ) ;
#7583=LINE ( 'NONE', #19411, #24340 ) ;
#7586=CARTESIAN_POINT ( 'NONE',  ( 38.31606138205700063, -6.758471399387619094, 56.13572720721855092 ) ) ;
#7588=( GEOMETRIC_REPRESENTATION_CONTEXT ( 3 ) GLOBAL_UNCERTAINTY_ASSIGNED_CONTEXT ( ( #20090 ) ) GLOBAL_UNIT_ASSIGNED_CONTEXT ( ( #6048, #17779, #12118 ) ) REPRESENTATION_CONTEXT ( 'NONE', 'WORKASPACE' ) );
#7591=ORIENTED_EDGE ( 'NONE', *, *, #20647, .F. ) ;
#7605=DIRECTION ( 'NONE',  ( 0.000000000000000000, -0.6568589528324746407, 0.7540134720837717852 ) ) ;
#7618=ORIENTED_EDGE ( 'NONE', *, *, #23820, .T. ) ;
#7632=( LENGTH_UNIT ( ) NAMED_UNIT ( * ) SI_UNIT ( .MILLI., .METRE. ) );
#7637=CARTESIAN_POINT ( 'NONE',  ( 33.31606138205700773, 7.043113989679085307, 66.83274420321491505 ) ) ;
#7639=VECTOR ( 'NONE', #11219, 1000.000000000000227 ) ;
#7682=DIRECTION ( 'NONE',  ( 1.000000000000000000, 0.000000000000000000, 0.000000000000000000 ) ) ;
#7685=VERTEX_POINT ( 'NONE', #15421 ) ;
#7698=ORIENTED_EDGE ( 'NONE', *, *, #9198, .T. ) ;
#7712=VERTEX_POINT ( 'NONE', #17874 ) ;
#7759=CARTESIAN_POINT ( 'NONE',  ( 35.31606138205700773, 3.296535697557906985, 65.33616386252352015 ) ) ;
#7762=CYLINDRICAL_SURFACE ( 'NONE', #19628, 0.7500000000000027756 ) ;
#7799=LINE ( 'NONE', #11299, #19449 ) ;
#7822=CIRCLE ( 'NONE', #22204, 1.249999999999998890 ) ;
#7824=FACE_OUTER_BOUND ( 'NONE', #13421, .T. ) ;
#7839=ORIENTED_EDGE ( 'NONE', *, *, #22859, .T. ) ;
#7844=EDGE_LOOP ( 'NONE', ( #19291, #398, #23880, #13400 ) ) ;
#7848=VECTOR ( 'NONE', #20771, 1000.000000000000227 ) ;
#7892=DIRECTION ( 'NONE',  ( 0.000000000000000000, -0.7540134720837687876, -0.6568589528324780824 ) ) ;
#7907=LINE ( 'NONE', #23474, #23835 ) ;
#7911=ORIENTED_EDGE ( 'NONE', *, *, #15703, .T. ) ;
#7926=EDGE_CURVE ( 'NONE', #19611, #17400, #4119, .T. ) ;
#7941=VERTEX_POINT ( 'NONE', #23707 ) ;
#7976=ORIENTED_EDGE ( 'NONE', *, *, #1979, .F. ) ;
#8016=VECTOR ( 'NONE', #23226, 1000.000000000000227 ) ;
#8018=LINE ( 'NONE', #8132, #51 ) ;
#8028=CARTESIAN_POINT ( 'NONE',  ( 38.31606138205700063, -4.399276463885007260, 59.51717649063222382 ) ) ;
#8086=DIRECTION ( 'NONE',  ( -1.000000000000000000, 0.000000000000000000, 0.000000000000000000 ) ) ;
#8113=DIRECTION ( 'NONE',  ( 1.000000000000000000, 0.000000000000000000, 0.000000000000000000 ) ) ;
#8115=ORIENTED_EDGE ( 'NONE', *, *, #23403, .T. ) ;
#8132=CARTESIAN_POINT ( 'NONE',  ( 35.31606138205700773, 3.099306811489555891, 65.29760936252343129 ) ) ;
#8147=EDGE_CURVE ( 'NONE', #16154, #20256, #6177, .T. ) ;
#8156=CARTESIAN_POINT ( 'NONE',  ( 33.31606138205700773, 3.536347952325769040, 64.10938348997790115 ) ) ;
#8165=AXIS2_PLACEMENT_3D ( 'NONE', #970, #19019, #1095 ) ;
#8166=VECTOR ( 'NONE', #5362, 1000.000000000000000 ) ;
#8178=EDGE_LOOP ( 'NONE', ( #14701, #6163, #4835, #18166 ) ) ;
#8197=EDGE_LOOP ( 'NONE', ( #8999, #19174, #8977, #17273 ) ) ;
#8200=VECTOR ( 'NONE', #3454, 1000.000000000000227 ) ;
#8207=LINE ( 'NONE', #10393, #2572 ) ;
#8218=VERTEX_POINT ( 'NONE', #2569 ) ;
#8222=CARTESIAN_POINT ( 'NONE',  ( 41.31606138205700063, 1.535676793533870210, 63.36117568837578062 ) ) ;
#8240=CARTESIAN_POINT ( 'NONE',  ( 41.31606138205700063, 1.207247317117632335, 63.73818242441765847 ) ) ;
#8252=ADVANCED_FACE ( 'NONE', ( #16236 ), #22158, .T. ) ;
#8283=DIRECTION ( 'NONE',  ( 0.000000000000000000, -0.7540134720837717852, -0.6568589528324746407 ) ) ;
#8307=EDGE_CURVE ( 'NONE', #5367, #4383, #13147, .T. ) ;
#8319=CARTESIAN_POINT ( 'NONE',  ( 32.31606138205700063, -20.55619265724211076, 44.11584019928223910 ) ) ;
#8362=AXIS2_PLACEMENT_3D ( 'NONE', #16256, #12165, #14215 ) ;
#8368=DIRECTION ( 'NONE',  ( 0.000000000000000000, 0.7540134720837717852, 0.6568589528324745297 ) ) ;
#8377=LINE ( 'NONE', #16219, #7441 ) ;
#8392=DIRECTION ( 'NONE',  ( 1.000000000000000000, 0.000000000000000000, 0.000000000000000000 ) ) ;
#8407=DIRECTION ( 'NONE',  ( 0.000000000000000000, -0.7540134720837697868, -0.6568589528324768612 ) ) ;
#8417=FACE_BOUND ( 'NONE', #25472, .T. ) ;
#8420=ORIENTED_EDGE ( 'NONE', *, *, #7580, .T. ) ;
#8428=VERTEX_POINT ( 'NONE', #3850 ) ;
#8436=DIRECTION ( 'NONE',  ( 1.000000000000000000, 0.000000000000000000, 0.000000000000000000 ) ) ;
#8441=DIRECTION ( 'NONE',  ( 1.000000000000000000, 0.000000000000000000, 0.000000000000000000 ) ) ;
#8445=CARTESIAN_POINT ( 'NONE',  ( 44.31606138205700063, -20.93319939328399926, 43.78741072286599945 ) ) ;
#8479=EDGE_CURVE ( 'NONE', #16267, #1997, #23425, .T. ) ;
#8489=DIRECTION ( 'NONE',  ( 0.000000000000000000, -0.6568589528324746407, 0.7540134720837716742 ) ) ;
#8493=EDGE_CURVE ( 'NONE', #13467, #973, #15568, .T. ) ;
#8510=DIRECTION ( 'NONE',  ( 0.000000000000000000, -0.6568589528324746407, 0.7540134720837716742 ) ) ;
#8515=DIRECTION ( 'NONE',  ( -1.000000000000000000, 0.000000000000000000, 0.000000000000000000 ) ) ;
#8540=FACE_OUTER_BOUND ( 'NONE', #14110, .T. ) ;
#8543=ORIENTED_EDGE ( 'NONE', *, *, #10450, .T. ) ;
#8550=CARTESIAN_POINT ( 'NONE',  ( 35.31606138205700773, 8.104266321858618838, 55.82104096753806033 ) ) ;
#8562=EDGE_CURVE ( 'NONE', #19118, #20855, #10163, .T. ) ;
#8576=VECTOR ( 'NONE', #22740, 1000.000000000000227 ) ;
#8585=FACE_OUTER_BOUND ( 'NONE', #1664, .T. ) ;
#8588=ORIENTED_EDGE ( 'NONE', *, *, #802, .F. ) ;
#8596=CARTESIAN_POINT ( 'NONE',  ( 32.31606138205700063, 10.06218483883314718, 67.80501292737497465 ) ) ;
#8599=DIRECTION ( 'NONE',  ( 0.000000000000000000, 0.7540134720837676774, 0.6568589528324791926 ) ) ;
#8616=PLANE ( 'NONE',  #23137 ) ;
#8618=CARTESIAN_POINT ( 'NONE',  ( 32.31606138205700063, -21.26162886970023536, 44.16441745890789150 ) ) ;
#8619=VECTOR ( 'NONE', #9392, 1000.000000000000000 ) ;
#8639=EDGE_CURVE ( 'NONE', #23124, #16518, #3677, .T. ) ;
#8673=PLANE ( 'NONE',  #23047 ) ;
#8692=VERTEX_POINT ( 'NONE', #24432 ) ;
#8753=DIRECTION ( 'NONE',  ( -1.000000000000000000, 0.000000000000000000, 0.000000000000000000 ) ) ;
#8758=ORIENTED_EDGE ( 'NONE', *, *, #19689, .F. ) ;
#8768=ADVANCED_FACE ( 'NONE', ( #20842 ), #14784, .F. ) ;
#8835=CARTESIAN_POINT ( 'NONE',  ( 33.31606138205700773, -21.26162886970023536, 44.16441745890789150 ) ) ;
#8839=ORIENTED_EDGE ( 'NONE', *, *, #114, .F. ) ;
#8840=FACE_OUTER_BOUND ( 'NONE', #20088, .T. ) ;
#8855=CARTESIAN_POINT ( 'NONE',  ( 33.31606138205700773, -21.26162886970023536, 44.16441745890789150 ) ) ;
#8864=ORIENTED_EDGE ( 'NONE', *, *, #13056, .F. ) ;
#8893=CARTESIAN_POINT ( 'NONE',  ( 44.31606138205700063, -20.55619265724211076, 44.11584019928223910 ) ) ;
#8923=ORIENTED_EDGE ( 'NONE', *, *, #24642, .T. ) ;
#8946=EDGE_CURVE ( 'NONE', #7685, #9479, #17551, .T. ) ;
#8947=DIRECTION ( 'NONE',  ( -1.000000000000000000, 0.000000000000000000, 0.000000000000000000 ) ) ;
#8950=ORIENTED_EDGE ( 'NONE', *, *, #758, .T. ) ;
#8958=DIRECTION ( 'NONE',  ( 0.000000000000000000, 0.1918498038142811835, -0.9814242980364923374 ) ) ;
#8959=ORIENTED_EDGE ( 'NONE', *, *, #15223, .F. ) ;
#8968=VERTEX_POINT ( 'NONE', #7759 ) ;
#8969=VERTEX_POINT ( 'NONE', #5569 ) ;
#8977=ORIENTED_EDGE ( 'NONE', *, *, #4369, .F. ) ;
#8999=ORIENTED_EDGE ( 'NONE', *, *, #6072, .F. ) ;
#9003=EDGE_CURVE ( 'NONE', #23360, #5934, #17910, .T. ) ;
#9075=CYLINDRICAL_SURFACE ( 'NONE', #21288, 1.249999999999998890 ) ;
#9112=VECTOR ( 'NONE', #8441, 1000.000000000000000 ) ;
#9118=FACE_OUTER_BOUND ( 'NONE', #18925, .T. ) ;
#9159=VECTOR ( 'NONE', #17493, 1000.000000000000227 ) ;
#9169=AXIS2_PLACEMENT_3D ( 'NONE', #17648, #15571, #9673 ) ;
#9180=EDGE_CURVE ( 'NONE', #21357, #7941, #381, .T. ) ;
#9198=EDGE_CURVE ( 'NONE', #10558, #19118, #17937, .T. ) ;
#9203=CARTESIAN_POINT ( 'NONE',  ( 33.31606138205700773, 7.043113989679085307, 66.83274420321491505 ) ) ;
#9204=VECTOR ( 'NONE', #2226, 1000.000000000000227 ) ;
#9209=DIRECTION ( 'NONE',  ( 1.000000000000000000, 0.000000000000000000, 0.000000000000000000 ) ) ;
#9215=ORIENTED_EDGE ( 'NONE', *, *, #18397, .F. ) ;
#9241=CIRCLE ( 'NONE', #14971, 1.500000000000001332 ) ;
#9244=DIRECTION ( 'NONE',  ( -1.000000000000000000, 0.000000000000000000, 0.000000000000000000 ) ) ;
#9252=FACE_OUTER_BOUND ( 'NONE', #432, .T. ) ;
#9280=ORIENTED_EDGE ( 'NONE', *, *, #5510, .F. ) ;
#9286=CARTESIAN_POINT ( 'NONE',  ( 0.000000000000000000, 0.000000000000000000, 0.000000000000000000 ) ) ;
#9288=CARTESIAN_POINT ( 'NONE',  ( 41.31606138205700063, 3.043703737701412226, 64.67489359404071081 ) ) ;
#9327=ORIENTED_EDGE ( 'NONE', *, *, #21529, .T. ) ;
#9353=EDGE_CURVE ( 'NONE', #20940, #7941, #24459, .T. ) ;
#9369=VERTEX_POINT ( 'NONE', #12648 ) ;
#9379=FACE_OUTER_BOUND ( 'NONE', #19717, .T. ) ;
#9392=DIRECTION ( 'NONE',  ( -1.000000000000000000, 0.000000000000000000, 0.000000000000000000 ) ) ;
#9394=PLANE ( 'NONE',  #17689 ) ;
#9406=DIRECTION ( 'NONE',  ( 0.000000000000000000, 0.6568589528324746407, -0.7540134720837716742 ) ) ;
#9422=AXIS2_PLACEMENT_3D ( 'NONE', #18225, #8436, #12812 ) ;
#9433=VERTEX_POINT ( 'NONE', #5790 ) ;
#9436=AXIS2_PLACEMENT_3D ( 'NONE', #11198, #20591, #20465 ) ;
#9449=ADVANCED_FACE ( 'NONE', ( #7470 ), #15320, .T. ) ;
#9479=VERTEX_POINT ( 'NONE', #3716 ) ;
#9513=ORIENTED_EDGE ( 'NONE', *, *, #8562, .T. ) ;
#9518=FACE_OUTER_BOUND ( 'NONE', #18771, .T. ) ;
#9526=CYLINDRICAL_SURFACE ( 'NONE', #17298, 0.7500000000000027756 ) ;
#9562=EDGE_CURVE ( 'NONE', #10558, #5367, #19192, .T. ) ;
#9566=FACE_OUTER_BOUND ( 'NONE', #4233, .T. ) ;
#9574=DIRECTION ( 'NONE',  ( -1.000000000000000000, 0.000000000000000000, 0.000000000000000000 ) ) ;
#9582=DIRECTION ( 'NONE',  ( 0.000000000000000000, 0.6568589528324747517, -0.7540134720837718962 ) ) ;
#9587=EDGE_CURVE ( 'NONE', #8968, #7941, #7112, .T. ) ;
#9590=ORIENTED_EDGE ( 'NONE', *, *, #2797, .T. ) ;
#9618=CARTESIAN_POINT ( 'NONE',  ( 41.31606138205700063, 3.536347952325769040, 64.10938348997790115 ) ) ;
#9634=ORIENTED_EDGE ( 'NONE', *, *, #11474, .T. ) ;
#9654=CARTESIAN_POINT ( 'NONE',  ( 32.31606138205700063, 10.62769494289597993, 68.29765714199933768 ) ) ;
#9673=DIRECTION ( 'NONE',  ( 0.000000000000000000, -0.7540134720837724513, -0.6568589528324737525 ) ) ;
#9696=DIRECTION ( 'NONE',  ( -1.000000000000000000, 0.000000000000000000, 0.000000000000000000 ) ) ;
#9699=FILL_AREA_STYLE ('',( #11886 ) ) ;
#9722=FACE_OUTER_BOUND ( 'NONE', #15910, .T. ) ;
#9726=ORIENTED_EDGE ( 'NONE', *, *, #3907, .F. ) ;
#9747=ORIENTED_EDGE ( 'NONE', *, *, #19638, .F. ) ;
#9774=ORIENTED_EDGE ( 'NONE', *, *, #8493, .F. ) ;
#9776=ORIENTED_EDGE ( 'NONE', *, *, #22042, .T. ) ;
#9779=VERTEX_POINT ( 'NONE', #12619 ) ;
#9788=VECTOR ( 'NONE', #5048, 1000.000000000000000 ) ;
#9807=AXIS2_PLACEMENT_3D ( 'NONE', #10777, #6902, #4726 ) ;
#9817=ADVANCED_FACE ( 'NONE', ( #12745 ), #8616, .T. ) ;
#9860=CIRCLE ( 'NONE', #20533, 0.7500000000000027756 ) ;
#9981=ORIENTED_EDGE ( 'NONE', *, *, #23886, .F. ) ;
#9983=LINE ( 'NONE', #6237, #3436 ) ;
#9986=CARTESIAN_POINT ( 'NONE',  ( 33.31606138205700773, 2.715274261285174351, 65.05190033008260286 ) ) ;
#9997=ORIENTED_EDGE ( 'NONE', *, *, #11134, .F. ) ;
#10022=CARTESIAN_POINT ( 'NONE',  ( 43.31606138205700063, 3.195231713396695650, 64.80689721350518084 ) ) ;
#10058=LINE ( 'NONE', #19444, #4921 ) ;
#10079=CARTESIAN_POINT ( 'NONE',  ( 33.31606138205700773, 2.715274261285174351, 65.05190033008260286 ) ) ;
#10080=ADVANCED_FACE ( 'NONE', ( #1383 ), #20178, .T. ) ;
#10091=AXIS2_PLACEMENT_3D ( 'NONE', #1812, #13428, #19468 ) ;
#10092=LINE ( 'NONE', #6216, #18808 ) ;
#10141=DIRECTION ( 'NONE',  ( 0.000000000000000000, 0.1918498038142811835, -0.9814242980364923374 ) ) ;
#10150=CARTESIAN_POINT ( 'NONE',  ( 33.31606138205700773, 9.119667998728431257, 66.98393923633439329 ) ) ;
#10157=ORIENTED_EDGE ( 'NONE', *, *, #21733, .T. ) ;
#10163=LINE ( 'NONE', #4245, #6975 ) ;
#10183=VECTOR ( 'NONE', #21164, 1000.000000000000000 ) ;
#10201=DIRECTION ( 'NONE',  ( 0.000000000000000000, 0.7540134720837717852, 0.6568589528324746407 ) ) ;
#10225=ADVANCED_FACE ( 'NONE', ( #21731 ), #6404, .F. ) ;
#10226=AXIS2_PLACEMENT_3D ( 'NONE', #9618, #9244, #25296 ) ;
#10233=EDGE_CURVE ( 'NONE', #20855, #14994, #8207, .T. ) ;
#10247=ORIENTED_EDGE ( 'NONE', *, *, #6762, .T. ) ;
#10254=ORIENTED_EDGE ( 'NONE', *, *, #21218, .T. ) ;
#10274=EDGE_CURVE ( 'NONE', #3043, #13140, #6019, .T. ) ;
#10281=ORIENTED_EDGE ( 'NONE', *, *, #758, .F. ) ;
#10313=CARTESIAN_POINT ( 'NONE',  ( 36.81606138205700063, -4.399276463885007260, 59.51717649063222382 ) ) ;
#10325=AXIS2_PLACEMENT_3D ( 'NONE', #2366, #16152, #13985 ) ;
#10386=AXIS2_PLACEMENT_3D ( 'NONE', #8156, #15999, #18929 ) ;
#10390=VERTEX_POINT ( 'NONE', #3150 ) ;
#10393=CARTESIAN_POINT ( 'NONE',  ( 41.81606138205700063, -21.26162886970023536, 44.16441745890789150 ) ) ;
#10396=AXIS2_PLACEMENT_3D ( 'NONE', #11859, #19310, #17388 ) ;
#10403=DIRECTION ( 'NONE',  ( -1.000000000000000000, 0.000000000000000000, 0.000000000000000000 ) ) ;
#10404=VECTOR ( 'NONE', #17350, 1000.000000000000000 ) ;
#10435=CARTESIAN_POINT ( 'NONE',  ( 32.31606138205700063, -20.93319939328399926, 43.78741072286599945 ) ) ;
#10450=EDGE_CURVE ( 'NONE', #25135, #23863, #7543, .T. ) ;
#10477=DIRECTION ( 'NONE',  ( 0.000000000000000000, 0.6568589528324747517, -0.7540134720837717852 ) ) ;
#10491=VECTOR ( 'NONE', #2242, 1000.000000000000227 ) ;
#10497=EDGE_CURVE ( 'NONE', #8968, #19348, #15388, .T. ) ;
#10534=DIRECTION ( 'NONE',  ( 0.000000000000000000, -0.6568589528324746407, 0.7540134720837717852 ) ) ;
#10554=LINE ( 'NONE', #8618, #17385 ) ;
#10558=VERTEX_POINT ( 'NONE', #11410 ) ;
#10595=EDGE_CURVE ( 'NONE', #1793, #6631, #17432, .T. ) ;
#10622=FACE_OUTER_BOUND ( 'NONE', #25362, .T. ) ;
#10645=EDGE_CURVE ( 'NONE', #16518, #14083, #9983, .T. ) ;
#10656=VECTOR ( 'NONE', #2616, 1000.000000000000000 ) ;
#10657=FACE_OUTER_BOUND ( 'NONE', #19627, .T. ) ;
#10691=DIRECTION ( 'NONE',  ( 0.000000000000000000, 0.6568589528324746407, -0.7540134720837716742 ) ) ;
#10701=FACE_OUTER_BOUND ( 'NONE', #2298, .T. ) ;
#10755=CARTESIAN_POINT ( 'NONE',  ( 38.31606138205700063, -6.758471399387619094, 56.13572720721855092 ) ) ;
#10768=PLANE ( 'NONE',  #22352 ) ;
#10772=CARTESIAN_POINT ( 'NONE',  ( 39.81606138205700063, -6.758471399387619094, 56.13572720721855092 ) ) ;
#10777=CARTESIAN_POINT ( 'NONE',  ( 32.31606138205700063, -20.93319939328399926, 43.78741072286599945 ) ) ;
#10779=DIRECTION ( 'NONE',  ( -0.000000000000000000, -0.7540134720837717852, -0.6568589528324747517 ) ) ;
#10819=VECTOR ( 'NONE', #18007, 1000.000000000000227 ) ;
#10863=VECTOR ( 'NONE', #12399, 1000.000000000000227 ) ;
#10881=ORIENTED_EDGE ( 'NONE', *, *, #22395, .F. ) ;
#10883=CARTESIAN_POINT ( 'NONE',  ( 34.81606138205700773, -21.26162886970023536, 44.16441745890789150 ) ) ;
#10892=VERTEX_POINT ( 'NONE', #6744 ) ;
#10916=DIRECTION ( 'NONE',  ( -1.000000000000000000, 0.000000000000000000, 0.000000000000000000 ) ) ;
#10963=VERTEX_POINT ( 'NONE', #22959 ) ;
#10977=EDGE_CURVE ( 'NONE', #24693, #24906, #13054, .T. ) ;
#10997=VECTOR ( 'NONE', #22070, 1000.000000000000227 ) ;
#11019=ADVANCED_FACE ( 'NONE', ( #6047 ), #5791, .F. ) ;
#11022=ORIENTED_EDGE ( 'NONE', *, *, #1859, .T. ) ;
#11039=ORIENTED_EDGE ( 'NONE', *, *, #4868, .F. ) ;
#11052=VECTOR ( 'NONE', #20948, 1000.000000000000000 ) ;
#11070=VECTOR ( 'NONE', #22544, 1000.000000000000227 ) ;
#11072=CIRCLE ( 'NONE', #14358, 1.500000000000001332 ) ;
#11079=ORIENTED_EDGE ( 'NONE', *, *, #13521, .F. ) ;
#11084=CIRCLE ( 'NONE', #6958, 0.7500000000000014433 ) ;
#11085=DIRECTION ( 'NONE',  ( -1.000000000000000000, 0.000000000000000000, 0.000000000000000000 ) ) ;
#11105=AXIS2_PLACEMENT_3D ( 'NONE', #6330, #8515, #24200 ) ;
#11115=VECTOR ( 'NONE', #16534, 1000.000000000000227 ) ;
#11132=DIRECTION ( 'NONE',  ( 1.000000000000000000, 0.000000000000000000, 0.000000000000000000 ) ) ;
#11134=EDGE_CURVE ( 'NONE', #20356, #21012, #10554, .T. ) ;
#11154=DIRECTION ( 'NONE',  ( 0.000000000000000000, 0.1918498038142821827, -0.9814242980364921154 ) ) ;
#11165=DIRECTION ( 'NONE',  ( 1.000000000000000000, 0.000000000000000000, 0.000000000000000000 ) ) ;
#11174=ORIENTED_EDGE ( 'NONE', *, *, #14150, .T. ) ;
#11177=CARTESIAN_POINT ( 'NONE',  ( 41.31606138205700063, 3.536347952325769040, 64.10938348997790115 ) ) ;
#11183=CARTESIAN_POINT ( 'NONE',  ( 35.31606138205700773, 8.104266321858618838, 55.82104096753806033 ) ) ;
#11192=DIRECTION ( 'NONE',  ( 0.000000000000000000, 0.6568589528324747517, -0.7540134720837717852 ) ) ;
#11193=DIRECTION ( 'NONE',  ( 0.000000000000000000, 0.9814242980364923374, 0.1918498038142812112 ) ) ;
#11197=CIRCLE ( 'NONE', #13652, 1.500000000000001332 ) ;
#11198=CARTESIAN_POINT ( 'NONE',  ( 38.31606138205700063, -1.383222575549920119, 62.14461230196212682 ) ) ;
#11202=FACE_OUTER_BOUND ( 'NONE', #14217, .T. ) ;
#11203=ORIENTED_EDGE ( 'NONE', *, *, #13650, .T. ) ;
#11219=DIRECTION ( 'NONE',  ( 0.000000000000000000, 0.7540134720837717852, 0.6568589528324746407 ) ) ;
#11234=LINE ( 'NONE', #1426, #18471 ) ;
#11272=ORIENTED_EDGE ( 'NONE', *, *, #22025, .T. ) ;
#11287=DIRECTION ( 'NONE',  ( 1.000000000000000000, 0.000000000000000000, 0.000000000000000000 ) ) ;
#11290=ORIENTED_EDGE ( 'NONE', *, *, #13650, .F. ) ;
#11295=EDGE_CURVE ( 'NONE', #20256, #4126, #20847, .T. ) ;
#11299=CARTESIAN_POINT ( 'NONE',  ( 33.31606138205700773, 7.282926244446933595, 65.60596383066929604 ) ) ;
#11302=AXIS2_PLACEMENT_3D ( 'NONE', #5096, #11287, #20679 ) ;
#11334=CARTESIAN_POINT ( 'NONE',  ( 32.31606138205700063, 9.733755362416909307, 68.18201966341686671 ) ) ;
#11350=DIRECTION ( 'NONE',  ( -1.000000000000000000, 0.000000000000000000, 0.000000000000000000 ) ) ;
#11364=ORIENTED_EDGE ( 'NONE', *, *, #13056, .T. ) ;
#11396=ORIENTED_EDGE ( 'NONE', *, *, #20647, .T. ) ;
#11405=CARTESIAN_POINT ( 'NONE',  ( 33.31606138205700773, 10.29926546647973851, 68.67466387804121553 ) ) ;
#11410=CARTESIAN_POINT ( 'NONE',  ( 34.81606138205700773, -8.868983839943650693, 54.29715396818559725 ) ) ;
#11415=ORIENTED_EDGE ( 'NONE', *, *, #10595, .T. ) ;
#11420=ORIENTED_EDGE ( 'NONE', *, *, #4114, .F. ) ;
#11439=ORIENTED_EDGE ( 'NONE', *, *, #19314, .T. ) ;
#11474=EDGE_CURVE ( 'NONE', #7685, #18044, #5764, .T. ) ;
#11478=EDGE_CURVE ( 'NONE', #9433, #2339, #7583, .T. ) ;
#11507=VECTOR ( 'NONE', #16210, 1000.000000000000227 ) ;
#11516=CARTESIAN_POINT ( 'NONE',  ( 33.31606138205700773, 3.296535697557910538, 65.33616386252352015 ) ) ;
#11529=ORIENTED_EDGE ( 'NONE', *, *, #9180, .F. ) ;
#11538=DIRECTION ( 'NONE',  ( 0.000000000000000000, 0.6568589528324746407, -0.7540134720837716742 ) ) ;
#11576=DIRECTION ( 'NONE',  ( 0.000000000000000000, 0.6568589528324745297, -0.7540134720837717852 ) ) ;
#11582=DIRECTION ( 'NONE',  ( -1.000000000000000000, 0.000000000000000000, 0.000000000000000000 ) ) ;
#11583=ORIENTED_EDGE ( 'NONE', *, *, #8479, .F. ) ;
#11587=AXIS2_PLACEMENT_3D ( 'NONE', #11183, #15797, #17737 ) ;
#11589=DIRECTION ( 'NONE',  ( -1.000000000000000000, 0.000000000000000000, 0.000000000000000000 ) ) ;
#11591=ORIENTED_EDGE ( 'NONE', *, *, #20261, .F. ) ;
#11599=SURFACE_SIDE_STYLE ('',( #23557 ) ) ;
#11623=PLANE ( 'NONE',  #19079 ) ;
#11627=EDGE_CURVE ( 'NONE', #6631, #12000, #14261, .T. ) ;
#11634=DIRECTION ( 'NONE',  ( 0.000000000000000000, 0.6568589528324747517, -0.7540134720837718962 ) ) ;
#11645=FACE_OUTER_BOUND ( 'NONE', #25201, .T. ) ;
#11651=CIRCLE ( 'NONE', #2573, 1.249999999999996891 ) ;
#11676=ORIENTED_EDGE ( 'NONE', *, *, #19005, .T. ) ;
#11692=ORIENTED_EDGE ( 'NONE', *, *, #17429, .T. ) ;
#11696=DIRECTION ( 'NONE',  ( 0.000000000000000000, -0.6568589528324746407, 0.7540134720837716742 ) ) ;
#11710=CARTESIAN_POINT ( 'NONE',  ( 33.31606138205700773, 7.187001342539796944, 66.09667597968754649 ) ) ;
#11715=EDGE_CURVE ( 'NONE', #16916, #1296, #13880, .T. ) ;
#11743=DIRECTION ( 'NONE',  ( 0.000000000000000000, 0.9814242980364923374, 0.1918498038142812112 ) ) ;
#11793=ORIENTED_EDGE ( 'NONE', *, *, #14530, .T. ) ;
#11811=CARTESIAN_POINT ( 'NONE',  ( 32.31606138205700063, 10.62769494289597993, 68.29765714199933768 ) ) ;
#11817=DIRECTION ( 'NONE',  ( 1.000000000000000000, 0.000000000000000000, 0.000000000000000000 ) ) ;
#11832=LINE ( 'NONE', #4348, #14321 ) ;
#11837=CARTESIAN_POINT ( 'NONE',  ( 44.31606138205700063, -21.26162886970023536, 44.16441745890789150 ) ) ;
#11846=DIRECTION ( 'NONE',  ( 0.000000000000000000, 0.7540134720837717852, 0.6568589528324746407 ) ) ;
#11859=CARTESIAN_POINT ( 'NONE',  ( 41.31606138205700063, 8.104266321858618838, 55.82104096753806033 ) ) ;
#11862=LINE ( 'NONE', #18159, #11507 ) ;
#11882=LINE ( 'NONE', #2440, #3009 ) ;
#11886=FILL_AREA_STYLE_COLOUR ( '', #13656 ) ;
#11902=ORIENTED_EDGE ( 'NONE', *, *, #333, .T. ) ;
#11939=EDGE_LOOP ( 'NONE', ( #23017, #6292, #17479, #2116 ) ) ;
#11953=EDGE_CURVE ( 'NONE', #22382, #981, #15513, .T. ) ;
#11967=CARTESIAN_POINT ( 'NONE',  ( 32.31606138205700063, 10.29926546647973851, 68.67466387804121553 ) ) ;
#11993=CARTESIAN_POINT ( 'NONE',  ( 38.31606138205700063, -1.054793099133682244, 61.76760556592023477 ) ) ;
#12000=VERTEX_POINT ( 'NONE', #19516 ) ;
#12035=FACE_OUTER_BOUND ( 'NONE', #2426, .T. ) ;
#12038=ORIENTED_EDGE ( 'NONE', *, *, #4522, .T. ) ;
#12044=EDGE_CURVE ( 'NONE', #18988, #12980, #7799, .T. ) ;
#12062=LINE ( 'NONE', #18234, #9112 ) ;
#12084=AXIS2_PLACEMENT_3D ( 'NONE', #8835, #16673, #24506 ) ;
#12118=( NAMED_UNIT ( * ) SI_UNIT ( $, .STERADIAN. ) SOLID_ANGLE_UNIT ( ) );
#12128=ORIENTED_EDGE ( 'NONE', *, *, #19966, .T. ) ;
#12130=PRODUCT_DEFINITION_CONTEXT ( 'detailed design', #6515, 'design' ) ;
#12147=DIRECTION ( 'NONE',  ( 0.000000000000000000, -0.6568589528324746407, 0.7540134720837717852 ) ) ;
#12165=DIRECTION ( 'NONE',  ( -1.000000000000000000, 0.000000000000000000, 0.000000000000000000 ) ) ;
#12178=EDGE_CURVE ( 'NONE', #3043, #16154, #21953, .T. ) ;
#12191=ORIENTED_EDGE ( 'NONE', *, *, #9180, .T. ) ;
#12212=LINE ( 'NONE', #11967, #20954 ) ;
#12216=LINE ( 'NONE', #10150, #6081 ) ;
#12217=EDGE_CURVE ( 'NONE', #24906, #21235, #17849, .T. ) ;
#12240=LINE ( 'NONE', #15955, #6551 ) ;
#12245=DIRECTION ( 'NONE',  ( 0.000000000000000000, -0.6568589528324746407, 0.7540134720837717852 ) ) ;
#12254=FACE_OUTER_BOUND ( 'NONE', #15491, .T. ) ;
#12269=LINE ( 'NONE', #4279, #20062 ) ;
#12286=DIRECTION ( 'NONE',  ( 0.000000000000000000, 0.1918498038142812112, -0.9814242980364923374 ) ) ;
#12328=ORIENTED_EDGE ( 'NONE', *, *, #20103, .T. ) ;
#12372=DIRECTION ( 'NONE',  ( 0.000000000000000000, 0.6568589528324746407, -0.7540134720837717852 ) ) ;
#12386=ORIENTED_EDGE ( 'NONE', *, *, #1756, .T. ) ;
#12390=CARTESIAN_POINT ( 'NONE',  ( 33.31606138205700773, 3.195231713396695650, 64.80689721350518084 ) ) ;
#12391=DIRECTION ( 'NONE',  ( -0.000000000000000000, -0.9814242980364923374, -0.1918498038142812112 ) ) ;
#12399=DIRECTION ( 'NONE',  ( 0.000000000000000000, 0.7540134720837717852, 0.6568589528324746407 ) ) ;
#12424=CARTESIAN_POINT ( 'NONE',  ( 43.31606138205700063, -20.88462213365835041, 44.49284693532412405 ) ) ;
#12426=DIRECTION ( 'NONE',  ( 0.000000000000000000, -0.6568589528324746407, 0.7540134720837716742 ) ) ;
#12436=VECTOR ( 'NONE', #22383, 1000.000000000000000 ) ;
#12471=DIRECTION ( 'NONE',  ( 0.000000000000000000, 0.6568589528324746407, -0.7540134720837717852 ) ) ;
#12472=CARTESIAN_POINT ( 'NONE',  ( 36.81606138205700063, -1.054793099133682244, 61.76760556592023477 ) ) ;
#12481=ORIENTED_EDGE ( 'NONE', *, *, #21218, .F. ) ;
#12482=DIRECTION ( 'NONE',  ( 0.000000000000000000, 0.9814242980364923374, 0.1918498038142812112 ) ) ;
#12491=CARTESIAN_POINT ( 'NONE',  ( 36.81606138205700063, -3.742417511052531509, 58.76316301854844681 ) ) ;
#12532=AXIS2_PLACEMENT_3D ( 'NONE', #2637, #6398, #698 ) ;
#12576=ORIENTED_EDGE ( 'NONE', *, *, #24774, .F. ) ;
#12619=CARTESIAN_POINT ( 'NONE',  ( 43.31606138205700063, 10.06218483883314718, 67.80501292737497465 ) ) ;
#12624=FACE_OUTER_BOUND ( 'NONE', #7844, .T. ) ;
#12629=UNCERTAINTY_MEASURE_WITH_UNIT (LENGTH_MEASURE( 1.000000000000000082E-05 ), #1909, 'distance_accuracy_value', 'NONE');
#12648=CARTESIAN_POINT ( 'NONE',  ( 36.81606138205700063, -7.086900875803856970, 56.51273394326043586 ) ) ;
#12689=LINE ( 'NONE', #5420, #20993 ) ;
#12698=FACE_OUTER_BOUND ( 'NONE', #18599, .T. ) ;
#12716=FACE_OUTER_BOUND ( 'NONE', #2111, .T. ) ;
#12718=VECTOR ( 'NONE', #21417, 1000.000000000000000 ) ;
#12740=AXIS2_PLACEMENT_3D ( 'NONE', #20119, #522, #8407 ) ;
#12745=FACE_OUTER_BOUND ( 'NONE', #2513, .T. ) ;
#12746=EDGE_CURVE ( 'NONE', #8428, #21357, #2825, .T. ) ;
#12759=ORIENTED_EDGE ( 'NONE', *, *, #1395, .T. ) ;
#12766=DIRECTION ( 'NONE',  ( 0.000000000000000000, 0.000000000000000000, 1.000000000000000000 ) ) ;
#12772=DIRECTION ( 'NONE',  ( 0.000000000000000000, 0.1918498038142811835, -0.9814242980364923374 ) ) ;
#12784=ORIENTED_EDGE ( 'NONE', *, *, #23886, .T. ) ;
#12812=DIRECTION ( 'NONE',  ( 0.000000000000000000, -0.7540134720837724513, -0.6568589528324737525 ) ) ;
#12861=DIRECTION ( 'NONE',  ( 0.000000000000000000, 0.6568589528324746407, -0.7540134720837716742 ) ) ;
#12872=EDGE_CURVE ( 'NONE', #13140, #20940, #24584, .T. ) ;
#12907=ORIENTED_EDGE ( 'NONE', *, *, #20364, .F. ) ;
#12921=ORIENTED_EDGE ( 'NONE', *, *, #23862, .F. ) ;
#12947=ORIENTED_EDGE ( 'NONE', *, *, #4697, .F. ) ;
#12954=CARTESIAN_POINT ( 'NONE',  ( 35.31606138205700773, 7.187001342539796944, 66.09667597968754649 ) ) ;
#12975=CARTESIAN_POINT ( 'NONE',  ( 41.81606138205700063, -2.300394311618905174, 46.75701924734788406 ) ) ;
#12979=CARTESIAN_POINT ( 'NONE',  ( 33.31606138205700773, 3.296535697557910538, 65.33616386252352015 ) ) ;
#12980=VERTEX_POINT ( 'NONE', #3214 ) ;
#13042=DIRECTION ( 'NONE',  ( -0.000000000000000000, -0.7540134720837717852, -0.6568589528324747517 ) ) ;
#13054=LINE ( 'NONE', #22835, #4686 ) ;
#13056=EDGE_CURVE ( 'NONE', #16916, #9369, #9241, .T. ) ;
#13071=EDGE_LOOP ( 'NONE', ( #19054, #5186, #6470, #12576 ) ) ;
#13072=DIRECTION ( 'NONE',  ( 0.000000000000000000, 0.6568589528324746407, -0.7540134720837717852 ) ) ;
#13083=VECTOR ( 'NONE', #7682, 1000.000000000000000 ) ;
#13094=CARTESIAN_POINT ( 'NONE',  ( 32.31606138205700063, 9.733755362416909307, 68.18201966341686671 ) ) ;
#13103=AXIS2_PLACEMENT_3D ( 'NONE', #5598, #25408, #17579 ) ;
#13117=DIRECTION ( 'NONE',  ( 1.000000000000000000, 0.000000000000000000, 0.000000000000000000 ) ) ;
#13123=CARTESIAN_POINT ( 'NONE',  ( 43.31606138205700063, 3.099306811489555891, 65.29760936252343129 ) ) ;
#13132=FACE_OUTER_BOUND ( 'NONE', #20973, .T. ) ;
#13140=VERTEX_POINT ( 'NONE', #8240 ) ;
#13141=DIRECTION ( 'NONE',  ( -1.000000000000000000, 0.000000000000000000, 0.000000000000000000 ) ) ;
#13147=LINE ( 'NONE', #16611, #11070 ) ;
#13192=LINE ( 'NONE', #23085, #20945 ) ;
#13197=CARTESIAN_POINT ( 'NONE',  ( 44.31606138205700063, -20.93319939328399926, 43.78741072286599945 ) ) ;
#13199=EDGE_LOOP ( 'NONE', ( #22865, #24018, #14044, #11396 ) ) ;
#13256=LINE ( 'NONE', #9654, #8200 ) ;
#13258=FACE_OUTER_BOUND ( 'NONE', #22182, .T. ) ;
#13260=LINE ( 'NONE', #21112, #23460 ) ;
#13274=ADVANCED_FACE ( 'NONE', ( #1093 ), #24788, .T. ) ;
#13279=PLANE ( 'NONE',  #3648 ) ;
#13287=EDGE_CURVE ( 'NONE', #23891, #6145, #20695, .T. ) ;
#13288=CARTESIAN_POINT ( 'NONE',  ( 33.31606138205700773, 7.535758204303438568, 66.26723409915207696 ) ) ;
#13306=SURFACE_SIDE_STYLE ('',( #25115 ) ) ;
#13310=CARTESIAN_POINT ( 'NONE',  ( 44.31606138205700063, 9.733755362416909307, 68.18201966341686671 ) ) ;
#13319=CARTESIAN_POINT ( 'NONE',  ( 32.31606138205700063, -21.26162886970023536, 44.16441745890789150 ) ) ;
#13327=ORIENTED_EDGE ( 'NONE', *, *, #9587, .F. ) ;
#13339=ADVANCED_FACE ( 'NONE', ( #4976 ), #18161, .T. ) ;
#13347=PLANE ( 'NONE',  #6049 ) ;
#13350=VECTOR ( 'NONE', #17863, 1000.000000000000000 ) ;
#13353=ORIENTED_EDGE ( 'NONE', *, *, #23403, .F. ) ;
#13400=ORIENTED_EDGE ( 'NONE', *, *, #23422, .F. ) ;
#13421=EDGE_LOOP ( 'NONE', ( #11692, #15282, #4455, #16423 ) ) ;
#13428=DIRECTION ( 'NONE',  ( -1.000000000000000000, 0.000000000000000000, 0.000000000000000000 ) ) ;
#13432=DIRECTION ( 'NONE',  ( 1.000000000000000000, 0.000000000000000000, 0.000000000000000000 ) ) ;
#13437=DIRECTION ( 'NONE',  ( 0.000000000000000000, 0.6568589528324747517, -0.7540134720837718962 ) ) ;
#13449=ORIENTED_EDGE ( 'NONE', *, *, #2457, .F. ) ;
#13455=ADVANCED_FACE ( 'NONE', ( #7824 ), #15670, .T. ) ;
#13458=EDGE_LOOP ( 'NONE', ( #21442, #16446, #9590, #11439 ) ) ;
#13467=VERTEX_POINT ( 'NONE', #23776 ) ;
#13485=CARTESIAN_POINT ( 'NONE',  ( 41.81606138205700063, -21.26162886970023536, 44.16441745890789150 ) ) ;
#13506=DIRECTION ( 'NONE',  ( 0.000000000000000000, -0.7540134720837687876, -0.6568589528324780824 ) ) ;
#13521=EDGE_CURVE ( 'NONE', #21012, #25135, #684, .T. ) ;
#13554=DIRECTION ( 'NONE',  ( 0.000000000000000000, -0.7540134720837717852, -0.6568589528324746407 ) ) ;
#13565=DIRECTION ( 'NONE',  ( -1.000000000000000000, 0.000000000000000000, 0.000000000000000000 ) ) ;
#13597=CARTESIAN_POINT ( 'NONE',  ( 33.31606138205700773, 7.611641054560886133, 65.67022133066943468 ) ) ;
#13600=DIRECTION ( 'NONE',  ( 1.000000000000000000, 0.000000000000000000, 0.000000000000000000 ) ) ;
#13622=VECTOR ( 'NONE', #5740, 1000.000000000000000 ) ;
#13626=CARTESIAN_POINT ( 'NONE',  ( 32.31606138205700063, 10.29926546647973851, 68.67466387804121553 ) ) ;
#13650=EDGE_CURVE ( 'NONE', #22400, #8692, #16035, .T. ) ;
#13652=AXIS2_PLACEMENT_3D ( 'NONE', #5645, #21361, #11589 ) ;
#13656=COLOUR_RGB ( '', 0.31764706, 0.68627451, 0.89019608) ;
#13673=ORIENTED_EDGE ( 'NONE', *, *, #24317, .F. ) ;
#13711=VECTOR ( 'NONE', #12471, 1000.000000000000227 ) ;
#13720=AXIS2_PLACEMENT_3D ( 'NONE', #15924, #21860, #18255 ) ;
#13762=CARTESIAN_POINT ( 'NONE',  ( 44.31606138205700063, -20.88462213365835041, 44.49284693532412405 ) ) ;
#13794=ORIENTED_EDGE ( 'NONE', *, *, #18059, .T. ) ;
#13835=ADVANCED_FACE ( 'NONE', ( #12698 ), #20538, .T. ) ;
#13836=PRODUCT_DEFINITION_SHAPE ( 'NONE', 'NONE',  #23307 ) ;
#13854=FACE_OUTER_BOUND ( 'NONE', #7077, .T. ) ;
#13880=LINE ( 'NONE', #4217, #13711 ) ;
#13881=CARTESIAN_POINT ( 'NONE',  ( 43.31606138205700063, -21.26162886970023536, 44.16441745890789150 ) ) ;
#13900=VECTOR ( 'NONE', #19248, 1000.000000000000000 ) ;
#13916=ORIENTED_EDGE ( 'NONE', *, *, #10450, .F. ) ;
#13919=AXIS2_PLACEMENT_3D ( 'NONE', #1091, #10779, #5112 ) ;
#13923=ORIENTED_EDGE ( 'NONE', *, *, #17754, .F. ) ;
#13933=( NAMED_UNIT ( * ) SI_UNIT ( $, .STERADIAN. ) SOLID_ANGLE_UNIT ( ) );
#13937=AXIS2_PLACEMENT_3D ( 'NONE', #22458, #13437, #7510 ) ;
#13950=CARTESIAN_POINT ( 'NONE',  ( 33.31606138205700773, 7.864187680719676443, 65.89022736311019912 ) ) ;
#13985=DIRECTION ( 'NONE',  ( 0.000000000000000000, 0.7540134720837717852, 0.6568589528324747517 ) ) ;
#13986=ORIENTED_EDGE ( 'NONE', *, *, #12178, .F. ) ;
#14016=ORIENTED_EDGE ( 'NONE', *, *, #15066, .T. ) ;
#14035=LINE ( 'NONE', #14169, #21775 ) ;
#14036=CARTESIAN_POINT ( 'NONE',  ( 38.31606138205700063, -7.086900875803856970, 56.51273394326043586 ) ) ;
#14044=ORIENTED_EDGE ( 'NONE', *, *, #5298, .F. ) ;
#14060=DIRECTION ( 'NONE',  ( 1.000000000000000000, 0.000000000000000000, 0.000000000000000000 ) ) ;
#14083=VERTEX_POINT ( 'NONE', #2592 ) ;
#14093=DIRECTION ( 'NONE',  ( 0.000000000000000000, 0.7540134720837717852, 0.6568589528324746407 ) ) ;
#14110=EDGE_LOOP ( 'NONE', ( #8959, #25300, #23341, #21082 ) ) ;
#14116=ADVANCED_FACE ( 'NONE', ( #12035 ), #6358, .T. ) ;
#14130=VERTEX_POINT ( 'NONE', #22184 ) ;
#14133=DIRECTION ( 'NONE',  ( -1.000000000000000000, 0.000000000000000000, 0.000000000000000000 ) ) ;
#14146=ORIENTED_EDGE ( 'NONE', *, *, #11474, .F. ) ;
#14150=EDGE_CURVE ( 'NONE', #21235, #8218, #20128, .T. ) ;
#14156=ADVANCED_FACE ( 'NONE', ( #23979, #532, #8417, #6474 ), #2088, .F. ) ;
#14169=CARTESIAN_POINT ( 'NONE',  ( 32.31606138205700063, -20.55619265724211076, 44.11584019928223910 ) ) ;
#14176=ADVANCED_FACE ( 'NONE', ( #6223 ), #17828, .T. ) ;
#14179=ORIENTED_EDGE ( 'NONE', *, *, #8493, .T. ) ;
#14197=DIRECTION ( 'NONE',  ( -1.000000000000000000, 0.000000000000000000, 0.000000000000000000 ) ) ;
#14215=DIRECTION ( 'NONE',  ( 0.000000000000000000, 0.7540134720837716742, 0.6568589528324746407 ) ) ;
#14217=EDGE_LOOP ( 'NONE', ( #3844, #6241, #815, #17508 ) ) ;
#14218=ORIENTED_EDGE ( 'NONE', *, *, #1395, .F. ) ;
#14231=CARTESIAN_POINT ( 'NONE',  ( 41.31606138205700063, 3.099306811489555891, 65.29760936252343129 ) ) ;
#14247=LINE ( 'NONE', #4587, #6217 ) ;
#14255=ORIENTED_EDGE ( 'NONE', *, *, #24798, .F. ) ;
#14261=LINE ( 'NONE', #10022, #10819 ) ;
#14269=LINE ( 'NONE', #20195, #7088 ) ;
#14286=DIRECTION ( 'NONE',  ( -0.000000000000000000, -0.7540134720837717852, -0.6568589528324747517 ) ) ;
#14306=CARTESIAN_POINT ( 'NONE',  ( 44.31606138205700063, -20.55619265724211076, 44.11584019928223910 ) ) ;
#14312=CARTESIAN_POINT ( 'NONE',  ( 34.81606138205700773, -2.300394311618905174, 46.75701924734788406 ) ) ;
#14321=VECTOR ( 'NONE', #8086, 1000.000000000000000 ) ;
#14358=AXIS2_PLACEMENT_3D ( 'NONE', #5580, #9582, #13565 ) ;
#14372=EDGE_CURVE ( 'NONE', #7712, #1793, #17638, .T. ) ;
#14403=VECTOR ( 'NONE', #20253, 1000.000000000000227 ) ;
#14469=CARTESIAN_POINT ( 'NONE',  ( 44.31606138205700063, 10.06218483883314718, 67.80501292737497465 ) ) ;
#14523=ORIENTED_EDGE ( 'NONE', *, *, #21529, .F. ) ;
#14526=CARTESIAN_POINT ( 'NONE',  ( 32.31606138205700063, 10.06218483883314718, 67.80501292737497465 ) ) ;
#14530=EDGE_CURVE ( 'NONE', #9369, #16916, #11197, .T. ) ;
#14545=ORIENTED_EDGE ( 'NONE', *, *, #19966, .F. ) ;
#14547=AXIS2_PLACEMENT_3D ( 'NONE', #17672, #9696, #23582 ) ;
#14555=EDGE_CURVE ( 'NONE', #7685, #18110, #2534, .T. ) ;
#14563=CARTESIAN_POINT ( 'NONE',  ( 41.31606138205700063, 2.715274261285174351, 65.05190033008260286 ) ) ;
#14685=PLANE ( 'NONE',  #2046 ) ;
#14691=EDGE_CURVE ( 'NONE', #15969, #981, #24050, .T. ) ;
#14701=ORIENTED_EDGE ( 'NONE', *, *, #10645, .T. ) ;
#14704=ORIENTED_EDGE ( 'NONE', *, *, #4232, .F. ) ;
#14758=CARTESIAN_POINT ( 'NONE',  ( 35.31606138205700773, 1.535676793533870210, 63.36117568837578062 ) ) ;
#14762=EDGE_CURVE ( 'NONE', #23854, #24510, #4990, .T. ) ;
#14763=DIRECTION ( 'NONE',  ( -0.000000000000000000, -0.7540134720837717852, -0.6568589528324747517 ) ) ;
#14774=ORIENTED_EDGE ( 'NONE', *, *, #23265, .F. ) ;
#14784=CYLINDRICAL_SURFACE ( 'NONE', #15423, 1.500000000000001332 ) ;
#14833=CARTESIAN_POINT ( 'NONE',  ( 38.31606138205700063, -4.070846987468769385, 59.14016975459033887 ) ) ;
#14834=AXIS2_PLACEMENT_3D ( 'NONE', #8893, #2937, #24448 ) ;
#14878=LINE ( 'NONE', #963, #8576 ) ;
#14933=VERTEX_POINT ( 'NONE', #19658 ) ;
#14965=( GEOMETRIC_REPRESENTATION_CONTEXT ( 3 ) GLOBAL_UNCERTAINTY_ASSIGNED_CONTEXT ( ( #12629 ) ) GLOBAL_UNIT_ASSIGNED_CONTEXT ( ( #1909, #19570, #17525 ) ) REPRESENTATION_CONTEXT ( 'NONE', 'WORKASPACE' ) );
#14971=AXIS2_PLACEMENT_3D ( 'NONE', #14036, #6182, #1912 ) ;
#14977=LINE ( 'NONE', #14469, #15145 ) ;
#14978=EDGE_CURVE ( 'NONE', #8428, #22767, #25436, .T. ) ;
#14987=DIRECTION ( 'NONE',  ( 0.000000000000000000, -0.6568589528324746407, 0.7540134720837717852 ) ) ;
#14994=VERTEX_POINT ( 'NONE', #13485 ) ;
#15001=FACE_OUTER_BOUND ( 'NONE', #4923, .T. ) ;
#15017=CARTESIAN_POINT ( 'NONE',  ( 33.31606138205700773, -21.26162886970023536, 44.16441745890789150 ) ) ;
#15026=DIRECTION ( 'NONE',  ( 0.000000000000000000, 0.7540134720837716742, 0.6568589528324746407 ) ) ;
#15049=ORIENTED_EDGE ( 'NONE', *, *, #20204, .T. ) ;
#15064=ADVANCED_FACE ( 'NONE', ( #3946 ), #3811, .T. ) ;
#15066=EDGE_CURVE ( 'NONE', #6859, #1793, #1870, .T. ) ;
#15080=DIRECTION ( 'NONE',  ( 0.000000000000000000, 0.7540134720837676774, 0.6568589528324791926 ) ) ;
#15084=ORIENTED_EDGE ( 'NONE', *, *, #20979, .F. ) ;
#15085=FACE_OUTER_BOUND ( 'NONE', #11939, .T. ) ;
#15134=CARTESIAN_POINT ( 'NONE',  ( 32.31606138205700063, -20.93319939328399926, 43.78741072286599945 ) ) ;
#15145=VECTOR ( 'NONE', #18720, 1000.000000000000000 ) ;
#15163=VECTOR ( 'NONE', #13600, 1000.000000000000000 ) ;
#15194=CIRCLE ( 'NONE', #4110, 0.7500000000000027756 ) ;
#15200=DIRECTION ( 'NONE',  ( 0.000000000000000000, 0.6568589528324746407, -0.7540134720837717852 ) ) ;
#15216=CARTESIAN_POINT ( 'NONE',  ( 41.31606138205700063, 14.21032488318011211, 61.14033482768515881 ) ) ;
#15223=EDGE_CURVE ( 'NONE', #22382, #16518, #20416, .T. ) ;
#15241=EDGE_LOOP ( 'NONE', ( #19448, #14523 ) ) ;
#15251=ORIENTED_EDGE ( 'NONE', *, *, #10233, .F. ) ;
#15282=ORIENTED_EDGE ( 'NONE', *, *, #10497, .T. ) ;
#15293=DIRECTION ( 'NONE',  ( -1.000000000000000000, 0.000000000000000000, 0.000000000000000000 ) ) ;
#15294=ADVANCED_FACE ( 'NONE', ( #15001 ), #10768, .T. ) ;
#15296=LINE ( 'NONE', #11710, #23373 ) ;
#15300=LINE ( 'NONE', #13762, #8619 ) ;
#15320=PLANE ( 'NONE',  #10396 ) ;
#15376=CARTESIAN_POINT ( 'NONE',  ( 39.81606138205700063, -3.742417511052531509, 58.76316301854844681 ) ) ;
#15384=ORIENTED_EDGE ( 'NONE', *, *, #8307, .F. ) ;
#15388=LINE ( 'NONE', #5354, #22357 ) ;
#15403=CARTESIAN_POINT ( 'NONE',  ( 39.81606138205700063, -0.7263636227174442572, 61.39059882987834982 ) ) ;
#15421=CARTESIAN_POINT ( 'NONE',  ( 41.31606138205700063, 7.864187680719676443, 65.89022736311019912 ) ) ;
#15423=AXIS2_PLACEMENT_3D ( 'NONE', #4996, #12861, #20716 ) ;
#15450=PRESENTATION_STYLE_ASSIGNMENT (( #2170 ) ) ;
#15451=CARTESIAN_POINT ( 'NONE',  ( 43.31606138205700063, 7.043113989679085307, 66.83274420321491505 ) ) ;
#15456=CARTESIAN_POINT ( 'NONE',  ( 35.31606138205700773, 1.207247317117632335, 63.73818242441765847 ) ) ;
#15491=EDGE_LOOP ( 'NONE', ( #2679, #13794, #7839, #17618 ) ) ;
#15510=FACE_OUTER_BOUND ( 'NONE', #22927, .T. ) ;
#15513=LINE ( 'NONE', #13597, #5062 ) ;
#15548=VECTOR ( 'NONE', #5388, 1000.000000000000227 ) ;
#15568=CIRCLE ( 'NONE', #25427, 1.500000000000001332 ) ;
#15571=DIRECTION ( 'NONE',  ( 1.000000000000000000, 0.000000000000000000, 0.000000000000000000 ) ) ;
#15578=CIRCLE ( 'NONE', #13937, 1.500000000000001332 ) ;
#15586=AXIS2_PLACEMENT_3D ( 'NONE', #11993, #19697, #484 ) ;
#15656=ORIENTED_EDGE ( 'NONE', *, *, #2457, .T. ) ;
#15670=PLANE ( 'NONE',  #7534 ) ;
#15673=AXIS2_PLACEMENT_3D ( 'NONE', #6500, #19776, #4064 ) ;
#15703=EDGE_CURVE ( 'NONE', #3936, #10892, #18089, .T. ) ;
#15778=LINE ( 'NONE', #23753, #15979 ) ;
#15797=DIRECTION ( 'NONE',  ( 1.000000000000000000, 0.000000000000000000, 0.000000000000000000 ) ) ;
#15830=SHAPE_REPRESENTATION_RELATIONSHIP ( 'NONE' , 'NONE' ,  #18165, #1241 ) ;
#15879=ORIENTED_EDGE ( 'NONE', *, *, #16250, .T. ) ;
#15910=EDGE_LOOP ( 'NONE', ( #21152, #18243, #12947, #22119 ) ) ;
#15924=CARTESIAN_POINT ( 'NONE',  ( 44.31606138205700063, -20.93319939328399926, 43.78741072286599945 ) ) ;
#15932=CARTESIAN_POINT ( 'NONE',  ( 43.31606138205700063, 7.282926244446933595, 65.60596383066929604 ) ) ;
#15946=ADVANCED_FACE ( 'NONE', ( #9566 ), #11623, .T. ) ;
#15948=VECTOR ( 'NONE', #23950, 1000.000000000000227 ) ;
#15949=DIRECTION ( 'NONE',  ( 0.000000000000000000, 0.6568589528324747517, -0.7540134720837718962 ) ) ;
#15955=CARTESIAN_POINT ( 'NONE',  ( 33.31606138205700773, 10.62769494289597993, 68.29765714199933768 ) ) ;
#15961=AXIS2_PLACEMENT_3D ( 'NONE', #22876, #5233, #24413 ) ;
#15969=VERTEX_POINT ( 'NONE', #17287 ) ;
#15979=VECTOR ( 'NONE', #21828, 1000.000000000000000 ) ;
#15992=ADVANCED_FACE ( 'NONE', ( #1549 ), #5946, .T. ) ;
#15999=DIRECTION ( 'NONE',  ( 1.000000000000000000, 0.000000000000000000, 0.000000000000000000 ) ) ;
#16020=VECTOR ( 'NONE', #16725, 1000.000000000000227 ) ;
#16030=ORIENTED_EDGE ( 'NONE', *, *, #17559, .T. ) ;
#16035=LINE ( 'NONE', #8445, #4298 ) ;
#16152=DIRECTION ( 'NONE',  ( 1.000000000000000000, 0.000000000000000000, 0.000000000000000000 ) ) ;
#16154=VERTEX_POINT ( 'NONE', #2311 ) ;
#16173=CYLINDRICAL_SURFACE ( 'NONE', #6864, 0.7500000000000027756 ) ;
#16179=ORIENTED_EDGE ( 'NONE', *, *, #14762, .F. ) ;
#16197=ORIENTED_EDGE ( 'NONE', *, *, #23406, .T. ) ;
#16204=CARTESIAN_POINT ( 'NONE',  ( 38.31606138205700063, -0.7263636227174442572, 61.39059882987834982 ) ) ;
#16209=STYLED_ITEM ( 'NONE', ( #15450 ), #1241 ) ;
#16210=DIRECTION ( 'NONE',  ( 0.000000000000000000, 0.6568589528324746407, -0.7540134720837717852 ) ) ;
#16219=CARTESIAN_POINT ( 'NONE',  ( 33.31606138205700773, 7.187001342539796944, 66.09667597968754649 ) ) ;
#16230=PLANE ( 'NONE',  #25403 ) ;
#16236=FACE_OUTER_BOUND ( 'NONE', #16688, .T. ) ;
#16250=EDGE_CURVE ( 'NONE', #3936, #8692, #11882, .T. ) ;
#16255=CARTESIAN_POINT ( 'NONE',  ( 44.31606138205700063, 10.29926546647973851, 68.67466387804121553 ) ) ;
#16256=CARTESIAN_POINT ( 'NONE',  ( 41.31606138205700063, 8.104266321858618838, 55.82104096753806033 ) ) ;
#16267=VERTEX_POINT ( 'NONE', #6071 ) ;
#16306=CARTESIAN_POINT ( 'NONE',  ( 41.31606138205700063, 7.043113989679085307, 66.83274420321491505 ) ) ;
#16307=ORIENTED_EDGE ( 'NONE', *, *, #18776, .T. ) ;
#16336=VERTEX_POINT ( 'NONE', #18552 ) ;
#16344=VECTOR ( 'NONE', #11576, 1000.000000000000000 ) ;
#16346=PLANE ( 'NONE',  #4875 ) ;
#16372=ORIENTED_EDGE ( 'NONE', *, *, #3453, .T. ) ;
#16423=ORIENTED_EDGE ( 'NONE', *, *, #6072, .T. ) ;
#16424=ORIENTED_EDGE ( 'NONE', *, *, #13287, .F. ) ;
#16441=LINE ( 'NONE', #2403, #20248 ) ;
#16446=ORIENTED_EDGE ( 'NONE', *, *, #14762, .T. ) ;
#16454=DIRECTION ( 'NONE',  ( 1.000000000000000000, 0.000000000000000000, 0.000000000000000000 ) ) ;
#16455=DIRECTION ( 'NONE',  ( 0.000000000000000000, 0.7540134720837717852, 0.6568589528324747517 ) ) ;
#16462=CARTESIAN_POINT ( 'NONE',  ( 38.31606138205700063, -7.415330352220093069, 56.88974067930232081 ) ) ;
#16487=ADVANCED_FACE ( 'NONE', ( #1641 ), #21366, .T. ) ;
#16503=LINE ( 'NONE', #909, #7848 ) ;
#16512=STYLED_ITEM ( 'NONE', ( #3499 ), #17413 ) ;
#16518=VERTEX_POINT ( 'NONE', #1518 ) ;
#16534=DIRECTION ( 'NONE',  ( 0.000000000000000000, -0.6568589528324746407, 0.7540134720837717852 ) ) ;
#16546=APPLICATION_CONTEXT ( 'automotive_design' ) ;
#16592=CARTESIAN_POINT ( 'NONE',  ( 34.81606138205700773, -9.197413316359888569, 54.67416070422748220 ) ) ;
#16611=CARTESIAN_POINT ( 'NONE',  ( 34.81606138205700773, -14.36460986495925241, 36.24727600202827915 ) ) ;
#16664=LINE ( 'NONE', #20660, #10656 ) ;
#16673=DIRECTION ( 'NONE',  ( -0.000000000000000000, -0.7540134720837717852, -0.6568589528324747517 ) ) ;
#16677=ORIENTED_EDGE ( 'NONE', *, *, #10274, .F. ) ;
#16688=EDGE_LOOP ( 'NONE', ( #17384, #1867, #18481, #24800 ) ) ;
#16696=ADVANCED_FACE ( 'NONE', ( #8585 ), #21628, .T. ) ;
#16709=CARTESIAN_POINT ( 'NONE',  ( 33.31606138205700773, 3.392460599465057403, 64.84545171350526971 ) ) ;
#16723=DIRECTION ( 'NONE',  ( 0.000000000000000000, 0.6568589528324746407, -0.7540134720837716742 ) ) ;
#16725=DIRECTION ( 'NONE',  ( 0.000000000000000000, 0.6568589528324746407, -0.7540134720837717852 ) ) ;
#16727=CARTESIAN_POINT ( 'NONE',  ( 39.81606138205700063, -4.070846987468769385, 59.14016975459033887 ) ) ;
#16823=ADVANCED_FACE ( 'NONE', ( #1471 ), #7277, .T. ) ;
#16848=VECTOR ( 'NONE', #7605, 1000.000000000000227 ) ;
#16859=AXIS2_PLACEMENT_3D ( 'NONE', #16462, #10691, #19050 ) ;
#16868=CARTESIAN_POINT ( 'NONE',  ( 34.81606138205700773, -20.93319939328399926, 43.78741072286599945 ) ) ;
#16916=VERTEX_POINT ( 'NONE', #7538 ) ;
#16969=VECTOR ( 'NONE', #4767, 1000.000000000000227 ) ;
#16977=CARTESIAN_POINT ( 'NONE',  ( 41.31606138205700063, 7.043113989679085307, 66.83274420321491505 ) ) ;
#16980=ORIENTED_EDGE ( 'NONE', *, *, #8307, .T. ) ;
#17000=LINE ( 'NONE', #25175, #4969 ) ;
#17031=ORIENTED_EDGE ( 'NONE', *, *, #8479, .T. ) ;
#17032=DIRECTION ( 'NONE',  ( 0.000000000000000000, 0.7540134720837716742, 0.6568589528324746407 ) ) ;
#17072=CARTESIAN_POINT ( 'NONE',  ( 33.31606138205700773, 7.283211578144648257, 66.04722806671131252 ) ) ;
#17101=EDGE_LOOP ( 'NONE', ( #6884, #3164, #10254, #23165 ) ) ;
#17102=ORIENTED_EDGE ( 'NONE', *, *, #20979, .T. ) ;
#17105=VERTEX_POINT ( 'NONE', #12424 ) ;
#17163=DIRECTION ( 'NONE',  ( 0.000000000000000000, -0.6568589528324746407, 0.7540134720837716742 ) ) ;
#17193=ORIENTED_EDGE ( 'NONE', *, *, #8147, .F. ) ;
#17240=CARTESIAN_POINT ( 'NONE',  ( 35.31606138205700773, 3.043703737701412226, 64.67489359404071081 ) ) ;
#17262=DIRECTION ( 'NONE',  ( 0.000000000000000000, 0.7540134720837716742, 0.6568589528324746407 ) ) ;
#17268=ORIENTED_EDGE ( 'NONE', *, *, #17754, .T. ) ;
#17273=ORIENTED_EDGE ( 'NONE', *, *, #9003, .T. ) ;
#17286=CARTESIAN_POINT ( 'NONE',  ( 43.31606138205700063, 3.392460599465057403, 64.84545171350526971 ) ) ;
#17287=CARTESIAN_POINT ( 'NONE',  ( 32.31606138205700063, 10.06218483883314718, 67.80501292737497465 ) ) ;
#17298=AXIS2_PLACEMENT_3D ( 'NONE', #88, #17632, #13506 ) ;
#17349=ORIENTED_EDGE ( 'NONE', *, *, #4522, .F. ) ;
#17350=DIRECTION ( 'NONE',  ( 0.000000000000000000, 0.6568589528324745297, -0.7540134720837717852 ) ) ;
#17373=ORIENTED_EDGE ( 'NONE', *, *, #11295, .F. ) ;
#17384=ORIENTED_EDGE ( 'NONE', *, *, #111, .F. ) ;
#17385=VECTOR ( 'NONE', #8368, 1000.000000000000000 ) ;
#17388=DIRECTION ( 'NONE',  ( 0.000000000000000000, 0.7540134720837716742, 0.6568589528324746407 ) ) ;
#17392=AXIS2_PLACEMENT_3D ( 'NONE', #20072, #18027, #8489 ) ;
#17400=VERTEX_POINT ( 'NONE', #4012 ) ;
#17413=MANIFOLD_SOLID_BREP ( 'NONE', #24953 ) ;
#17429=EDGE_CURVE ( 'NONE', #5934, #8968, #8018, .T. ) ;
#17432=CIRCLE ( 'NONE', #23994, 0.7500000000000041078 ) ;
#17457=CYLINDRICAL_SURFACE ( 'NONE', #13103, 1.249999999999998890 ) ;
#17476=ORIENTED_EDGE ( 'NONE', *, *, #20550, .F. ) ;
#17479=ORIENTED_EDGE ( 'NONE', *, *, #14555, .F. ) ;
#17480=CARTESIAN_POINT ( 'NONE',  ( 41.31606138205700063, 7.535758204303438568, 66.26723409915207696 ) ) ;
#17493=DIRECTION ( 'NONE',  ( 0.000000000000000000, -0.6568589528324746407, 0.7540134720837717852 ) ) ;
#17508=ORIENTED_EDGE ( 'NONE', *, *, #24798, .T. ) ;
#17523=EDGE_CURVE ( 'NONE', #18244, #16267, #634, .T. ) ;
#17524=CARTESIAN_POINT ( 'NONE',  ( 32.31606138205700063, 10.06218483883314718, 67.80501292737497465 ) ) ;
#17525=( NAMED_UNIT ( * ) SI_UNIT ( $, .STERADIAN. ) SOLID_ANGLE_UNIT ( ) );
#17534=ORIENTED_EDGE ( 'NONE', *, *, #23422, .T. ) ;
#17549=( NAMED_UNIT ( * ) PLANE_ANGLE_UNIT ( ) SI_UNIT ( $, .RADIAN. ) );
#17551=LINE ( 'NONE', #1554, #18803 ) ;
#17559=EDGE_CURVE ( 'NONE', #3043, #6859, #20485, .T. ) ;
#17579=DIRECTION ( 'NONE',  ( 0.000000000000000000, -0.7540134720837725624, -0.6568589528324736415 ) ) ;
#17604=EDGE_LOOP ( 'NONE', ( #13449, #11290, #23185, #17981 ) ) ;
#17618=ORIENTED_EDGE ( 'NONE', *, *, #3730, .T. ) ;
#17630=DIRECTION ( 'NONE',  ( 0.000000000000000000, 0.6568589528324747517, -0.7540134720837718962 ) ) ;
#17632=DIRECTION ( 'NONE',  ( 1.000000000000000000, 0.000000000000000000, 0.000000000000000000 ) ) ;
#17633=ORIENTED_EDGE ( 'NONE', *, *, #12044, .T. ) ;
#17638=LINE ( 'NONE', #17899, #1710 ) ;
#17648=CARTESIAN_POINT ( 'NONE',  ( 35.31606138205700773, 3.536347952325769040, 64.10938348997790115 ) ) ;
#17654=VECTOR ( 'NONE', #14987, 1000.000000000000227 ) ;
#17672=CARTESIAN_POINT ( 'NONE',  ( 41.31606138205700063, 8.104266321858618838, 55.82104096753806033 ) ) ;
#17674=DIRECTION ( 'NONE',  ( 0.000000000000000000, 0.6568589528324747517, -0.7540134720837718962 ) ) ;
#17689=AXIS2_PLACEMENT_3D ( 'NONE', #1265, #20984, #1127 ) ;
#17709=EDGE_CURVE ( 'NONE', #24693, #8218, #14269, .T. ) ;
#17710=AXIS2_PLACEMENT_3D ( 'NONE', #12390, #12772, #11085 ) ;
#17732=ORIENTED_EDGE ( 'NONE', *, *, #12178, .T. ) ;
#17737=DIRECTION ( 'NONE',  ( 0.000000000000000000, -0.6568589528324746407, 0.7540134720837716742 ) ) ;
#17746=DIRECTION ( 'NONE',  ( 0.000000000000000000, -0.7540134720837717852, -0.6568589528324746407 ) ) ;
#17752=PRODUCT ( 'Pusher Link Lever', 'Pusher Link Lever', '', ( #3382 ) ) ;
#17754=EDGE_CURVE ( 'NONE', #21009, #18244, #16441, .T. ) ;
#17779=( NAMED_UNIT ( * ) PLANE_ANGLE_UNIT ( ) SI_UNIT ( $, .RADIAN. ) );
#17782=AXIS2_PLACEMENT_3D ( 'NONE', #4854, #10916, #15026 ) ;
#17790=VERTEX_POINT ( 'NONE', #8222 ) ;
#17818=DIRECTION ( 'NONE',  ( 1.000000000000000000, 0.000000000000000000, 0.000000000000000000 ) ) ;
#17828=CYLINDRICAL_SURFACE ( 'NONE', #10386, 1.249999999999998668 ) ;
#17849=LINE ( 'NONE', #14231, #7537 ) ;
#17854=ORIENTED_EDGE ( 'NONE', *, *, #25471, .T. ) ;
#17858=ADVANCED_FACE ( 'NONE', ( #9252 ), #6918, .T. ) ;
#17863=DIRECTION ( 'NONE',  ( 0.000000000000000000, 0.6568589528324745297, -0.7540134720837717852 ) ) ;
#17869=CARTESIAN_POINT ( 'NONE',  ( 33.31606138205700773, 3.043703737701412226, 64.67489359404071081 ) ) ;
#17874=CARTESIAN_POINT ( 'NONE',  ( 43.31606138205700063, -20.55619265724211076, 44.11584019928223910 ) ) ;
#17899=CARTESIAN_POINT ( 'NONE',  ( 43.31606138205700063, -20.93319939328399926, 43.78741072286599945 ) ) ;
#17910=CIRCLE ( 'NONE', #10091, 0.7500000000000021094 ) ;
#17926=AXIS2_PLACEMENT_3D ( 'NONE', #4761, #13141, #7214 ) ;
#17928=DIRECTION ( 'NONE',  ( 1.000000000000000000, 0.000000000000000000, 0.000000000000000000 ) ) ;
#17937=LINE ( 'NONE', #14312, #18361 ) ;
#17980=EDGE_LOOP ( 'NONE', ( #3521, #3304, #7467, #9776 ) ) ;
#17981=ORIENTED_EDGE ( 'NONE', *, *, #21733, .F. ) ;
#18001=ORIENTED_EDGE ( 'NONE', *, *, #18059, .F. ) ;
#18007=DIRECTION ( 'NONE',  ( 0.000000000000000000, 0.9814242980364923374, 0.1918498038142812112 ) ) ;
#18017=EDGE_LOOP ( 'NONE', ( #7976, #3669, #1208, #8115, #11676, #1245, #21304, #25027, #21948, #25391, #19702, #1719 ) ) ;
#18027=DIRECTION ( 'NONE',  ( 1.000000000000000000, 0.000000000000000000, 0.000000000000000000 ) ) ;
#18044=VERTEX_POINT ( 'NONE', #60 ) ;
#18046=CIRCLE ( 'NONE', #10226, 1.249999999999998890 ) ;
#18050=ORIENTED_EDGE ( 'NONE', *, *, #13287, .T. ) ;
#18059=EDGE_CURVE ( 'NONE', #2190, #15969, #23127, .T. ) ;
#18089=LINE ( 'NONE', #18337, #9204 ) ;
#18105=EDGE_CURVE ( 'NONE', #23863, #5367, #23506, .T. ) ;
#18110=VERTEX_POINT ( 'NONE', #17480 ) ;
#18159=CARTESIAN_POINT ( 'NONE',  ( 33.31606138205700773, 2.715274261285174351, 65.05190033008260286 ) ) ;
#18160=EDGE_CURVE ( 'NONE', #18110, #9433, #23377, .T. ) ;
#18161=PLANE ( 'NONE',  #23963 ) ;
#18165=SHAPE_REPRESENTATION ( 'Pusher Link Lever', ( #2000 ), #7588 ) ;
#18166=ORIENTED_EDGE ( 'NONE', *, *, #15223, .T. ) ;
#18216=ORIENTED_EDGE ( 'NONE', *, *, #23406, .F. ) ;
#18225=CARTESIAN_POINT ( 'NONE',  ( 33.31606138205700773, 3.536347952325769040, 64.10938348997790115 ) ) ;
#18234=CARTESIAN_POINT ( 'NONE',  ( 33.31606138205700773, 7.187001342539796944, 66.09667597968754649 ) ) ;
#18243=ORIENTED_EDGE ( 'NONE', *, *, #4369, .T. ) ;
#18244=VERTEX_POINT ( 'NONE', #24174 ) ;
#18250=VECTOR ( 'NONE', #17746, 1000.000000000000227 ) ;
#18255=DIRECTION ( 'NONE',  ( 0.000000000000000000, -0.6568589528324746407, 0.7540134720837716742 ) ) ;
#18337=CARTESIAN_POINT ( 'NONE',  ( 41.81606138205700063, -20.93319939328399926, 43.78741072286599945 ) ) ;
#18361=VECTOR ( 'NONE', #12147, 1000.000000000000227 ) ;
#18369=CARTESIAN_POINT ( 'NONE',  ( 33.31606138205700773, 3.536347952325769040, 64.10938348997790115 ) ) ;
#18372=EDGE_LOOP ( 'NONE', ( #12907, #2430 ) ) ;
#18375=ADVANCED_FACE ( 'NONE', ( #995, #18655, #7582, #9518 ), #7194, .T. ) ;
#18388=VECTOR ( 'NONE', #13554, 1000.000000000000227 ) ;
#18392=ORIENTED_EDGE ( 'NONE', *, *, #15703, .F. ) ;
#18393=VERTEX_POINT ( 'NONE', #13626 ) ;
#18397=EDGE_CURVE ( 'NONE', #17105, #7712, #21102, .T. ) ;
#18424=DIRECTION ( 'NONE',  ( -1.000000000000000000, 0.000000000000000000, 0.000000000000000000 ) ) ;
#18451=LINE ( 'NONE', #16255, #14403 ) ;
#18471=VECTOR ( 'NONE', #23810, 1000.000000000000227 ) ;
#18481=ORIENTED_EDGE ( 'NONE', *, *, #19713, .T. ) ;
#18525=DIRECTION ( 'NONE',  ( 0.000000000000000000, 0.7540134720837676774, 0.6568589528324791926 ) ) ;
#18551=FACE_OUTER_BOUND ( 'NONE', #8178, .T. ) ;
#18552=CARTESIAN_POINT ( 'NONE',  ( 43.31606138205700063, 7.535758204303438568, 66.26723409915207696 ) ) ;
#18599=EDGE_LOOP ( 'NONE', ( #5346, #23030, #15879, #15656 ) ) ;
#18612=VECTOR ( 'NONE', #11193, 1000.000000000000227 ) ;
#18620=ORIENTED_EDGE ( 'NONE', *, *, #18660, .F. ) ;
#18641=ORIENTED_EDGE ( 'NONE', *, *, #18397, .T. ) ;
#18655=FACE_BOUND ( 'NONE', #18372, .T. ) ;
#18660=EDGE_CURVE ( 'NONE', #10892, #10558, #11832, .T. ) ;
#18691=CARTESIAN_POINT ( 'NONE',  ( 33.31606138205700773, -21.26162886970023536, 44.16441745890789150 ) ) ;
#18720=DIRECTION ( 'NONE',  ( -1.000000000000000000, 0.000000000000000000, 0.000000000000000000 ) ) ;
#18771=EDGE_LOOP ( 'NONE', ( #21327, #19816, #6227, #13916, #20051, #16197, #22632, #12038, #12128, #6539, #14016, #1896, #5783, #11203, #19276, #7911 ) ) ;
#18776=EDGE_CURVE ( 'NONE', #22473, #7941, #14878, .T. ) ;
#18784=FACE_OUTER_BOUND ( 'NONE', #24014, .T. ) ;
#18786=CYLINDRICAL_SURFACE ( 'NONE', #22584, 1.500000000000001332 ) ;
#18789=LINE ( 'NONE', #5393, #16020 ) ;
#18803=VECTOR ( 'NONE', #21541, 1000.000000000000000 ) ;
#18808=VECTOR ( 'NONE', #4159, 1000.000000000000000 ) ;
#18854=ADVANCED_FACE ( 'NONE', ( #12716 ), #2892, .T. ) ;
#18865=VERTEX_POINT ( 'NONE', #14758 ) ;
#18874=VECTOR ( 'NONE', #5788, 1000.000000000000227 ) ;
#18924=CARTESIAN_POINT ( 'NONE',  ( 33.31606138205700773, 3.296535697557910538, 65.33616386252352015 ) ) ;
#18925=EDGE_LOOP ( 'NONE', ( #16179, #7591, #746, #17102 ) ) ;
#18929=DIRECTION ( 'NONE',  ( 0.000000000000000000, -0.7540134720837724513, -0.6568589528324737525 ) ) ;
#18988=VERTEX_POINT ( 'NONE', #20981 ) ;
#19005=EDGE_CURVE ( 'NONE', #16336, #8969, #1260, .T. ) ;
#19009=ORIENTED_EDGE ( 'NONE', *, *, #11627, .T. ) ;
#19019=DIRECTION ( 'NONE',  ( -1.000000000000000000, 0.000000000000000000, 0.000000000000000000 ) ) ;
#19027=CARTESIAN_POINT ( 'NONE',  ( 43.31606138205700063, 7.187001342539796944, 66.09667597968754649 ) ) ;
#19029=EDGE_LOOP ( 'NONE', ( #19009, #8950, #17373, #12759 ) ) ;
#19041=CARTESIAN_POINT ( 'NONE',  ( 43.31606138205700063, -20.55619265724211076, 44.11584019928223910 ) ) ;
#19048=CARTESIAN_POINT ( 'NONE',  ( 35.31606138205700773, 7.864187680719676443, 65.89022736311019912 ) ) ;
#19050=DIRECTION ( 'NONE',  ( -1.000000000000000000, 0.000000000000000000, 0.000000000000000000 ) ) ;
#19054=ORIENTED_EDGE ( 'NONE', *, *, #19713, .F. ) ;
#19079=AXIS2_PLACEMENT_3D ( 'NONE', #25373, #3496, #17163 ) ;
#19087=AXIS2_PLACEMENT_3D ( 'NONE', #17524, #23555, #4120 ) ;
#19118=VERTEX_POINT ( 'NONE', #16592 ) ;
#19133=FACE_OUTER_BOUND ( 'NONE', #13071, .T. ) ;
#19143=LINE ( 'NONE', #1479, #15163 ) ;
#19154=VERTEX_POINT ( 'NONE', #24438 ) ;
#19169=ADVANCED_FACE ( 'NONE', ( #18784 ), #1123, .T. ) ;
#19174=ORIENTED_EDGE ( 'NONE', *, *, #2081, .F. ) ;
#19188=EDGE_CURVE ( 'NONE', #12980, #19348, #23023, .T. ) ;
#19192=LINE ( 'NONE', #1524, #512 ) ;
#19199=DIRECTION ( 'NONE',  ( 0.000000000000000000, 0.7540134720837717852, 0.6568589528324746407 ) ) ;
#19248=DIRECTION ( 'NONE',  ( 1.000000000000000000, 0.000000000000000000, 0.000000000000000000 ) ) ;
#19253=DIRECTION ( 'NONE',  ( 0.000000000000000000, -0.7540134720837717852, -0.6568589528324746407 ) ) ;
#19259=LINE ( 'NONE', #13094, #8166 ) ;
#19269=EDGE_LOOP ( 'NONE', ( #21085, #14704, #6259, #8420 ) ) ;
#19276=ORIENTED_EDGE ( 'NONE', *, *, #16250, .F. ) ;
#19291=ORIENTED_EDGE ( 'NONE', *, *, #3353, .F. ) ;
#19292=CARTESIAN_POINT ( 'NONE',  ( 33.31606138205700773, 2.715274261285174351, 65.05190033008260286 ) ) ;
#19310=DIRECTION ( 'NONE',  ( -1.000000000000000000, 0.000000000000000000, 0.000000000000000000 ) ) ;
#19314=EDGE_CURVE ( 'NONE', #23124, #18988, #15296, .T. ) ;
#19332=ORIENTED_EDGE ( 'NONE', *, *, #3907, .T. ) ;
#19348=VERTEX_POINT ( 'NONE', #4095 ) ;
#19408=ORIENTED_EDGE ( 'NONE', *, *, #22431, .T. ) ;
#19411=CARTESIAN_POINT ( 'NONE',  ( 33.31606138205700773, 8.791238522312193382, 67.36094597237627113 ) ) ;
#19413=CARTESIAN_POINT ( 'NONE',  ( 35.31606138205700773, 3.195231713396695650, 64.80689721350518084 ) ) ;
#19430=VECTOR ( 'NONE', #25454, 1000.000000000000227 ) ;
#19444=CARTESIAN_POINT ( 'NONE',  ( 33.31606138205700773, 3.195231713396695650, 64.80689721350518084 ) ) ;
#19448=ORIENTED_EDGE ( 'NONE', *, *, #22490, .F. ) ;
#19449=VECTOR ( 'NONE', #5605, 1000.000000000000000 ) ;
#19456=ORIENTED_EDGE ( 'NONE', *, *, #22431, .F. ) ;
#19468=DIRECTION ( 'NONE',  ( 0.000000000000000000, -0.7540134720837682325, -0.6568589528324786375 ) ) ;
#19482=DIRECTION ( 'NONE',  ( -1.000000000000000000, 0.000000000000000000, 0.000000000000000000 ) ) ;
#19509=ORIENTED_EDGE ( 'NONE', *, *, #9562, .F. ) ;
#19516=CARTESIAN_POINT ( 'NONE',  ( 43.31606138205700063, 7.282926244446933595, 65.60596383066929604 ) ) ;
#19527=DIRECTION ( 'NONE',  ( 0.000000000000000000, 0.7540134720837717852, 0.6568589528324746407 ) ) ;
#19534=DIRECTION ( 'NONE',  ( 1.000000000000000000, 0.000000000000000000, 0.000000000000000000 ) ) ;
#19546=ADVANCED_FACE ( 'NONE', ( #10657 ), #708, .T. ) ;
#19570=( NAMED_UNIT ( * ) PLANE_ANGLE_UNIT ( ) SI_UNIT ( $, .RADIAN. ) );
#19611=VERTEX_POINT ( 'NONE', #12472 ) ;
#19627=EDGE_LOOP ( 'NONE', ( #11591, #21280, #17031, #4721 ) ) ;
#19628=AXIS2_PLACEMENT_3D ( 'NONE', #7637, #13432, #7892 ) ;
#19638=EDGE_CURVE ( 'NONE', #24147, #14083, #19259, .T. ) ;
#19649=EDGE_CURVE ( 'NONE', #4383, #19118, #5606, .T. ) ;
#19658=CARTESIAN_POINT ( 'NONE',  ( 36.81606138205700063, -4.070846987468769385, 59.14016975459033887 ) ) ;
#19659=ORIENTED_EDGE ( 'NONE', *, *, #19649, .F. ) ;
#19689=EDGE_CURVE ( 'NONE', #20356, #4383, #3420, .T. ) ;
#19697=DIRECTION ( 'NONE',  ( 0.000000000000000000, 0.6568589528324747517, -0.7540134720837718962 ) ) ;
#19702=ORIENTED_EDGE ( 'NONE', *, *, #10645, .F. ) ;
#19713=EDGE_CURVE ( 'NONE', #8218, #12000, #19143, .T. ) ;
#19717=EDGE_LOOP ( 'NONE', ( #23873, #17476, #4790, #6094 ) ) ;
#19719=EDGE_CURVE ( 'NONE', #1997, #8969, #22872, .T. ) ;
#19736=CARTESIAN_POINT ( 'NONE',  ( 35.31606138205700773, 3.536347952325769040, 64.10938348997790115 ) ) ;
#19747=AXIS2_PLACEMENT_3D ( 'NONE', #6208, #21794, #4152 ) ;
#19766=DIRECTION ( 'NONE',  ( 1.000000000000000000, 0.000000000000000000, 0.000000000000000000 ) ) ;
#19776=DIRECTION ( 'NONE',  ( 0.000000000000000000, -0.7540134720837717852, -0.6568589528324745297 ) ) ;
#19777=ORIENTED_EDGE ( 'NONE', *, *, #8562, .F. ) ;
#19787=CARTESIAN_POINT ( 'NONE',  ( 43.31606138205700063, 7.535758204303438568, 66.26723409915207696 ) ) ;
#19791=EDGE_CURVE ( 'NONE', #3043, #24906, #18046, .T. ) ;
#19804=DIRECTION ( 'NONE',  ( 0.000000000000000000, 0.7540134720837717852, 0.6568589528324746407 ) ) ;
#19807=CARTESIAN_POINT ( 'NONE',  ( 32.31606138205700063, -20.93319939328399926, 43.78741072286599945 ) ) ;
#19816=ORIENTED_EDGE ( 'NONE', *, *, #9562, .T. ) ;
#19835=ORIENTED_EDGE ( 'NONE', *, *, #19791, .F. ) ;
#19897=VECTOR ( 'NONE', #19253, 1000.000000000000227 ) ;
#19909=PLANE ( 'NONE',  #15673 ) ;
#19938=PRODUCT_DEFINITION_FORMATION_WITH_SPECIFIED_SOURCE ( 'ANY', '', #17752, .NOT_KNOWN. ) ;
#19966=EDGE_CURVE ( 'NONE', #18865, #17790, #15778, .T. ) ;
#20051=ORIENTED_EDGE ( 'NONE', *, *, #3502, .T. ) ;
#20062=VECTOR ( 'NONE', #20113, 1000.000000000000227 ) ;
#20072=CARTESIAN_POINT ( 'NONE',  ( 43.31606138205700063, 3.043703737701412226, 64.67489359404071081 ) ) ;
#20076=AXIS2_PLACEMENT_3D ( 'NONE', #1709, #11538, #5855 ) ;
#20087=DIRECTION ( 'NONE',  ( 1.000000000000000000, 0.000000000000000000, 0.000000000000000000 ) ) ;
#20088=EDGE_LOOP ( 'NONE', ( #1611, #14255, #5986, #12784 ) ) ;
#20090=UNCERTAINTY_MEASURE_WITH_UNIT (LENGTH_MEASURE( 1.000000000000000082E-05 ), #6048, 'distance_accuracy_value', 'NONE');
#20103=EDGE_CURVE ( 'NONE', #21012, #8428, #16664, .T. ) ;
#20105=AXIS2_PLACEMENT_3D ( 'NONE', #5847, #2563, #4515 ) ;
#20113=DIRECTION ( 'NONE',  ( 0.000000000000000000, 0.9814242980364923374, 0.1918498038142812112 ) ) ;
#20119=CARTESIAN_POINT ( 'NONE',  ( 33.31606138205700773, 3.536347952325769040, 64.10938348997790115 ) ) ;
#20128=LINE ( 'NONE', #159, #2178 ) ;
#20137=ADVANCED_FACE ( 'NONE', ( #10622 ), #6749, .T. ) ;
#20143=AXIS2_PLACEMENT_3D ( 'NONE', #7586, #17630, #11582 ) ;
#20178=PLANE ( 'NONE',  #13720 ) ;
#20190=EDGE_CURVE ( 'NONE', #6145, #7242, #15578, .T. ) ;
#20195=CARTESIAN_POINT ( 'NONE',  ( 41.31606138205700063, 3.195231713396695650, 64.80689721350518084 ) ) ;
#20204=EDGE_CURVE ( 'NONE', #24906, #20256, #5701, .T. ) ;
#20211=DIRECTION ( 'NONE',  ( -1.000000000000000000, 0.000000000000000000, 0.000000000000000000 ) ) ;
#20248=VECTOR ( 'NONE', #6290, 1000.000000000000227 ) ;
#20253=DIRECTION ( 'NONE',  ( 0.000000000000000000, 0.7540134720837717852, 0.6568589528324746407 ) ) ;
#20256=VERTEX_POINT ( 'NONE', #22966 ) ;
#20261=EDGE_CURVE ( 'NONE', #9779, #8969, #25261, .T. ) ;
#20276=EDGE_CURVE ( 'NONE', #23854, #19348, #13192, .T. ) ;
#20309=ORIENTED_EDGE ( 'NONE', *, *, #8147, .T. ) ;
#20329=ORIENTED_EDGE ( 'NONE', *, *, #22859, .F. ) ;
#20356=VERTEX_POINT ( 'NONE', #13319 ) ;
#20357=LINE ( 'NONE', #14306, #3921 ) ;
#20364=EDGE_CURVE ( 'NONE', #7242, #6145, #11072, .T. ) ;
#20369=CARTESIAN_POINT ( 'NONE',  ( 41.31606138205700063, 1.207247317117632335, 63.73818242441765847 ) ) ;
#20386=ORIENTED_EDGE ( 'NONE', *, *, #3719, .F. ) ;
#20416=LINE ( 'NONE', #6767, #24343 ) ;
#20427=ADVANCED_FACE ( 'NONE', ( #21924 ), #25387, .F. ) ;
#20465=DIRECTION ( 'NONE',  ( -1.000000000000000000, 0.000000000000000000, 0.000000000000000000 ) ) ;
#20476=AXIS2_PLACEMENT_3D ( 'NONE', #5141, #20849, #23277 ) ;
#20485=LINE ( 'NONE', #4895, #16969 ) ;
#20533=AXIS2_PLACEMENT_3D ( 'NONE', #19736, #17818, #149 ) ;
#20538=PLANE ( 'NONE',  #12084 ) ;
#20545=CARTESIAN_POINT ( 'NONE',  ( 33.31606138205700773, 3.195231713396695650, 64.80689721350518084 ) ) ;
#20550=EDGE_CURVE ( 'NONE', #19348, #22473, #9860, .T. ) ;
#20585=DIRECTION ( 'NONE',  ( 0.000000000000000000, 0.6568589528324746407, -0.7540134720837716742 ) ) ;
#20591=DIRECTION ( 'NONE',  ( 0.000000000000000000, 0.6568589528324746407, -0.7540134720837716742 ) ) ;
#20597=DIRECTION ( 'NONE',  ( 0.000000000000000000, -0.6568589528324746407, 0.7540134720837716742 ) ) ;
#20598=ORIENTED_EDGE ( 'NONE', *, *, #13521, .T. ) ;
#20607=PLANE ( 'NONE',  #14834 ) ;
#20619=CARTESIAN_POINT ( 'NONE',  ( 35.31606138205700773, 1.207247317117632335, 63.73818242441765847 ) ) ;
#20647=EDGE_CURVE ( 'NONE', #19154, #23854, #4900, .T. ) ;
#20660=CARTESIAN_POINT ( 'NONE',  ( 32.31606138205700063, -20.88462213365835041, 44.49284693532412405 ) ) ;
#20679=DIRECTION ( 'NONE',  ( 0.000000000000000000, -0.6568589528324746407, 0.7540134720837716742 ) ) ;
#20695=LINE ( 'NONE', #3291, #1808 ) ;
#20716=DIRECTION ( 'NONE',  ( -1.000000000000000000, 0.000000000000000000, 0.000000000000000000 ) ) ;
#20731=DIRECTION ( 'NONE',  ( 1.000000000000000000, 0.000000000000000000, 0.000000000000000000 ) ) ;
#20771=DIRECTION ( 'NONE',  ( 0.000000000000000000, 0.6568589528324746407, -0.7540134720837717852 ) ) ;
#20774=CARTESIAN_POINT ( 'NONE',  ( 33.31606138205700773, 3.392460599465057403, 64.84545171350526971 ) ) ;
#20842=FACE_OUTER_BOUND ( 'NONE', #4545, .T. ) ;
#20847=LINE ( 'NONE', #13123, #18612 ) ;
#20849=DIRECTION ( 'NONE',  ( -1.000000000000000000, 0.000000000000000000, 0.000000000000000000 ) ) ;
#20855=VERTEX_POINT ( 'NONE', #5173 ) ;
#20869=CIRCLE ( 'NONE', #25367, 1.249999999999997780 ) ;
#20933=ORIENTED_EDGE ( 'NONE', *, *, #14372, .T. ) ;
#20940=VERTEX_POINT ( 'NONE', #15456 ) ;
#20945=VECTOR ( 'NONE', #9209, 1000.000000000000000 ) ;
#20948=DIRECTION ( 'NONE',  ( -1.000000000000000000, 0.000000000000000000, 0.000000000000000000 ) ) ;
#20949=EDGE_CURVE ( 'NONE', #23854, #18988, #10058, .T. ) ;
#20954=VECTOR ( 'NONE', #4477, 1000.000000000000227 ) ;
#20971=EDGE_LOOP ( 'NONE', ( #9774, #8588 ) ) ;
#20973=EDGE_LOOP ( 'NONE', ( #18641, #20933, #5289, #20386 ) ) ;
#20978=VECTOR ( 'NONE', #10534, 1000.000000000000227 ) ;
#20979=EDGE_CURVE ( 'NONE', #21357, #24510, #7822, .T. ) ;
#20981=CARTESIAN_POINT ( 'NONE',  ( 33.31606138205700773, 7.282926244446933595, 65.60596383066929604 ) ) ;
#20984=DIRECTION ( 'NONE',  ( -1.000000000000000000, 0.000000000000000000, 0.000000000000000000 ) ) ;
#20993=VECTOR ( 'NONE', #15200, 1000.000000000000227 ) ;
#21009=VERTEX_POINT ( 'NONE', #25355 ) ;
#21012=VERTEX_POINT ( 'NONE', #21639 ) ;
#21015=CARTESIAN_POINT ( 'NONE',  ( 43.31606138205700063, 7.043113989679085307, 66.83274420321491505 ) ) ;
#21048=( GEOMETRIC_REPRESENTATION_CONTEXT ( 3 ) GLOBAL_UNCERTAINTY_ASSIGNED_CONTEXT ( ( #22087 ) ) GLOBAL_UNIT_ASSIGNED_CONTEXT ( ( #7632, #17549, #13933 ) ) REPRESENTATION_CONTEXT ( 'NONE', 'WORKASPACE' ) );
#21076=ADVANCED_FACE ( 'NONE', ( #22269 ), #2677, .F. ) ;
#21077=ADVANCED_FACE ( 'NONE', ( #13258 ), #9394, .T. ) ;
#21082=ORIENTED_EDGE ( 'NONE', *, *, #8639, .T. ) ;
#21085=ORIENTED_EDGE ( 'NONE', *, *, #11478, .T. ) ;
#21088=DIRECTION ( 'NONE',  ( -1.000000000000000000, 0.000000000000000000, 0.000000000000000000 ) ) ;
#21102=LINE ( 'NONE', #19041, #16344 ) ;
#21112=CARTESIAN_POINT ( 'NONE',  ( 35.31606138205700773, 8.104266321858618838, 55.82104096753806033 ) ) ;
#21113=ORIENTED_EDGE ( 'NONE', *, *, #19649, .T. ) ;
#21152=ORIENTED_EDGE ( 'NONE', *, *, #1979, .T. ) ;
#21163=ORIENTED_EDGE ( 'NONE', *, *, #9353, .T. ) ;
#21164=DIRECTION ( 'NONE',  ( 1.000000000000000000, 0.000000000000000000, 0.000000000000000000 ) ) ;
#21196=DIRECTION ( 'NONE',  ( 0.000000000000000000, 0.7540134720837716742, 0.6568589528324746407 ) ) ;
#21218=EDGE_CURVE ( 'NONE', #9369, #10963, #18789, .T. ) ;
#21235=VERTEX_POINT ( 'NONE', #3064 ) ;
#21269=AXIS2_PLACEMENT_3D ( 'NONE', #13197, #19482, #1827 ) ;
#21280=ORIENTED_EDGE ( 'NONE', *, *, #1859, .F. ) ;
#21288=AXIS2_PLACEMENT_3D ( 'NONE', #9203, #4937, #3245 ) ;
#21304=ORIENTED_EDGE ( 'NONE', *, *, #4695, .T. ) ;
#21307=VECTOR ( 'NONE', #18424, 1000.000000000000000 ) ;
#21319=CARTESIAN_POINT ( 'NONE',  ( 34.81606138205700773, -21.26162886970023536, 44.16441745890789150 ) ) ;
#21327=ORIENTED_EDGE ( 'NONE', *, *, #18660, .T. ) ;
#21328=CARTESIAN_POINT ( 'NONE',  ( 33.31606138205700773, -20.93319939328399926, 43.78741072286599945 ) ) ;
#21346=CARTESIAN_POINT ( 'NONE',  ( 41.31606138205700063, 7.611641054560886133, 65.67022133066943468 ) ) ;
#21355=CARTESIAN_POINT ( 'NONE',  ( 41.31606138205700063, -20.93319939328399926, 43.78741072286599945 ) ) ;
#21357=VERTEX_POINT ( 'NONE', #19292 ) ;
#21361=DIRECTION ( 'NONE',  ( 0.000000000000000000, 0.6568589528324747517, -0.7540134720837718962 ) ) ;
#21366=PLANE ( 'NONE',  #1401 ) ;
#21378=FACE_OUTER_BOUND ( 'NONE', #17980, .T. ) ;
#21386=AXIS2_PLACEMENT_3D ( 'NONE', #13950, #22054, #6095 ) ;
#21410=AXIS2_PLACEMENT_3D ( 'NONE', #24941, #3065, #20597 ) ;
#21412=CARTESIAN_POINT ( 'NONE',  ( 38.31606138205700063, -4.070846987468769385, 59.14016975459033887 ) ) ;
#21417=DIRECTION ( 'NONE',  ( 1.000000000000000000, 0.000000000000000000, 0.000000000000000000 ) ) ;
#21442=ORIENTED_EDGE ( 'NONE', *, *, #20949, .F. ) ;
#21458=ORIENTED_EDGE ( 'NONE', *, *, #22708, .T. ) ;
#21463=ORIENTED_EDGE ( 'NONE', *, *, #20204, .F. ) ;
#21466=EDGE_LOOP ( 'NONE', ( #4967, #15049, #24885, #12921 ) ) ;
#21502=CARTESIAN_POINT ( 'NONE',  ( 41.81606138205700063, -2.300394311618905174, 46.75701924734788406 ) ) ;
#21529=EDGE_CURVE ( 'NONE', #1296, #10963, #5639, .T. ) ;
#21537=ADVANCED_FACE ( 'NONE', ( #11645 ), #23215, .F. ) ;
#21541=DIRECTION ( 'NONE',  ( 1.000000000000000000, 0.000000000000000000, 0.000000000000000000 ) ) ;
#21547=ADVANCED_FACE ( 'NONE', ( #25389 ), #5582, .F. ) ;
#21564=CARTESIAN_POINT ( 'NONE',  ( 35.31606138205700773, 7.282926244446937147, 65.60596383066929604 ) ) ;
#21573=ORIENTED_EDGE ( 'NONE', *, *, #7580, .F. ) ;
#21576=CARTESIAN_POINT ( 'NONE',  ( 33.31606138205700773, 7.611641054560886133, 65.67022133066943468 ) ) ;
#21589=CARTESIAN_POINT ( 'NONE',  ( 33.31606138205700773, 7.864187680719676443, 65.89022736311019912 ) ) ;
#21628=PLANE ( 'NONE',  #12532 ) ;
#21639=CARTESIAN_POINT ( 'NONE',  ( 32.31606138205700063, -20.88462213365835041, 44.49284693532412405 ) ) ;
#21662=LINE ( 'NONE', #4016, #10183 ) ;
#21680=DIRECTION ( 'NONE',  ( 0.000000000000000000, 0.7540134720837716742, 0.6568589528324746407 ) ) ;
#21690=LINE ( 'NONE', #4042, #3200 ) ;
#21710=ORIENTED_EDGE ( 'NONE', *, *, #3719, .T. ) ;
#21731=FACE_OUTER_BOUND ( 'NONE', #21466, .T. ) ;
#21733=EDGE_CURVE ( 'NONE', #22403, #14130, #10092, .T. ) ;
#21775=VECTOR ( 'NONE', #22015, 1000.000000000000000 ) ;
#21794=DIRECTION ( 'NONE',  ( 1.000000000000000000, 0.000000000000000000, 0.000000000000000000 ) ) ;
#21799=DIRECTION ( 'NONE',  ( -1.000000000000000000, 0.000000000000000000, 0.000000000000000000 ) ) ;
#21807=CARTESIAN_POINT ( 'NONE',  ( 35.31606138205700773, 7.611641054560886133, 65.67022133066943468 ) ) ;
#21828=DIRECTION ( 'NONE',  ( 1.000000000000000000, 0.000000000000000000, 0.000000000000000000 ) ) ;
#21860=DIRECTION ( 'NONE',  ( 1.000000000000000000, 0.000000000000000000, 0.000000000000000000 ) ) ;
#21883=PLANE ( 'NONE',  #17392 ) ;
#21924=FACE_OUTER_BOUND ( 'NONE', #24794, .T. ) ;
#21947=ORIENTED_EDGE ( 'NONE', *, *, #3353, .T. ) ;
#21948=ORIENTED_EDGE ( 'NONE', *, *, #3730, .F. ) ;
#21950=LINE ( 'NONE', #4181, #10997 ) ;
#21953=LINE ( 'NONE', #9986, #5896 ) ;
#21977=COLOUR_RGB ( '', 0.31764706, 0.68627451, 0.89019608) ;
#21997=DIRECTION ( 'NONE',  ( 1.000000000000000000, 0.000000000000000000, 0.000000000000000000 ) ) ;
#22015=DIRECTION ( 'NONE',  ( 1.000000000000000000, 0.000000000000000000, 0.000000000000000000 ) ) ;
#22021=LINE ( 'NONE', #2554, #1253 ) ;
#22025=EDGE_CURVE ( 'NONE', #4126, #16336, #11084, .T. ) ;
#22030=CARTESIAN_POINT ( 'NONE',  ( 32.31606138205700063, -20.93319939328399926, 43.78741072286599945 ) ) ;
#22031=ORIENTED_EDGE ( 'NONE', *, *, #5849, .T. ) ;
#22037=CARTESIAN_POINT ( 'NONE',  ( 44.31606138205700063, 10.62769494289597993, 68.29765714199933768 ) ) ;
#22042=EDGE_CURVE ( 'NONE', #16336, #9479, #11234, .T. ) ;
#22054=DIRECTION ( 'NONE',  ( -1.000000000000000000, 0.000000000000000000, 0.000000000000000000 ) ) ;
#22070=DIRECTION ( 'NONE',  ( 0.000000000000000000, -0.6568589528324746407, 0.7540134720837717852 ) ) ;
#22087=UNCERTAINTY_MEASURE_WITH_UNIT (LENGTH_MEASURE( 1.000000000000000082E-05 ), #7632, 'distance_accuracy_value', 'NONE');
#22102=FACE_OUTER_BOUND ( 'NONE', #13199, .T. ) ;
#22119=ORIENTED_EDGE ( 'NONE', *, *, #4232, .T. ) ;
#22147=VECTOR ( 'NONE', #11165, 1000.000000000000000 ) ;
#22158=PLANE ( 'NONE',  #17710 ) ;
#22166=EDGE_CURVE ( 'NONE', #2190, #18244, #12240, .T. ) ;
#22182=EDGE_LOOP ( 'NONE', ( #12386, #15251, #9726, #18392 ) ) ;
#22184=CARTESIAN_POINT ( 'NONE',  ( 44.31606138205700063, -20.88462213365835041, 44.49284693532412405 ) ) ;
#22204=AXIS2_PLACEMENT_3D ( 'NONE', #5666, #5930, #1916 ) ;
#22220=VERTEX_POINT ( 'NONE', #19048 ) ;
#22229=DIRECTION ( 'NONE',  ( 0.000000000000000000, -0.7540134720837687876, -0.6568589528324780824 ) ) ;
#22269=FACE_OUTER_BOUND ( 'NONE', #718, .T. ) ;
#22300=ADVANCED_FACE ( 'NONE', ( #7065 ), #18786, .F. ) ;
#22303=ADVANCED_FACE ( 'NONE', ( #12624 ), #4876, .F. ) ;
#22342=ORIENTED_EDGE ( 'NONE', *, *, #4114, .T. ) ;
#22352=AXIS2_PLACEMENT_3D ( 'NONE', #20545, #8958, #6886 ) ;
#22357=VECTOR ( 'NONE', #11154, 1000.000000000000227 ) ;
#22382=VERTEX_POINT ( 'NONE', #7201 ) ;
#22383=DIRECTION ( 'NONE',  ( 1.000000000000000000, 0.000000000000000000, 0.000000000000000000 ) ) ;
#22395=EDGE_CURVE ( 'NONE', #18393, #2190, #13256, .T. ) ;
#22400=VERTEX_POINT ( 'NONE', #25196 ) ;
#22403=VERTEX_POINT ( 'NONE', #11837 ) ;
#22404=EDGE_LOOP ( 'NONE', ( #14774, #11415, #14218, #17193 ) ) ;
#22431=EDGE_CURVE ( 'NONE', #14130, #17105, #15300, .T. ) ;
#22458=CARTESIAN_POINT ( 'NONE',  ( 38.31606138205700063, -3.742417511052531509, 58.76316301854844681 ) ) ;
#22459=LINE ( 'NONE', #13288, #3292 ) ;
#22465=ORIENTED_EDGE ( 'NONE', *, *, #2785, .T. ) ;
#22473=VERTEX_POINT ( 'NONE', #17240 ) ;
#22490=EDGE_CURVE ( 'NONE', #10963, #1296, #2420, .T. ) ;
#22513=DIRECTION ( 'NONE',  ( 1.000000000000000000, 0.000000000000000000, 0.000000000000000000 ) ) ;
#22516=CIRCLE ( 'NONE', #3586, 1.500000000000001332 ) ;
#22537=DIRECTION ( 'NONE',  ( 1.000000000000000000, 0.000000000000000000, 0.000000000000000000 ) ) ;
#22544=DIRECTION ( 'NONE',  ( 0.000000000000000000, -0.6568589528324746407, 0.7540134720837717852 ) ) ;
#22584=AXIS2_PLACEMENT_3D ( 'NONE', #3322, #16723, #8753 ) ;
#22632=ORIENTED_EDGE ( 'NONE', *, *, #5298, .T. ) ;
#22642=AXIS2_PLACEMENT_3D ( 'NONE', #16306, #21997, #8599 ) ;
#22663=LINE ( 'NONE', #6951, #21307 ) ;
#22708=EDGE_CURVE ( 'NONE', #23863, #20356, #2398, .T. ) ;
#22733=CARTESIAN_POINT ( 'NONE',  ( 43.31606138205700063, 3.296535697557910538, 65.33616386252352015 ) ) ;
#22734=ORIENTED_EDGE ( 'NONE', *, *, #12044, .F. ) ;
#22740=DIRECTION ( 'NONE',  ( 0.000000000000000000, -0.6568589528324746407, 0.7540134720837717852 ) ) ;
#22748=PLANE ( 'NONE',  #8165 ) ;
#22758=EDGE_LOOP ( 'NONE', ( #23884, #16980, #8758, #1404 ) ) ;
#22767=VERTEX_POINT ( 'NONE', #85 ) ;
#22785=VECTOR ( 'NONE', #893, 1000.000000000000000 ) ;
#22797=ORIENTED_EDGE ( 'NONE', *, *, #20190, .T. ) ;
#22821=DIRECTION ( 'NONE',  ( -1.000000000000000000, 0.000000000000000000, 0.000000000000000000 ) ) ;
#22834=ORIENTED_EDGE ( 'NONE', *, *, #20364, .T. ) ;
#22835=CARTESIAN_POINT ( 'NONE',  ( 41.31606138205700063, 3.392460599465057403, 64.84545171350526971 ) ) ;
#22859=EDGE_CURVE ( 'NONE', #15969, #24147, #2897, .T. ) ;
#22865=ORIENTED_EDGE ( 'NONE', *, *, #20276, .T. ) ;
#22872=LINE ( 'NONE', #5230, #11052 ) ;
#22876=CARTESIAN_POINT ( 'NONE',  ( 38.31606138205700063, -0.7263636227174442572, 61.39059882987834982 ) ) ;
#22891=CARTESIAN_POINT ( 'NONE',  ( 33.31606138205700773, 7.043113989679085307, 66.83274420321491505 ) ) ;
#22927=EDGE_LOOP ( 'NONE', ( #25109, #6922, #23673, #3663, #3403, #18001, #24097, #1655, #11022, #9280, #7287, #9634 ) ) ;
#22959=CARTESIAN_POINT ( 'NONE',  ( 36.81606138205700063, -6.758471399387619094, 56.13572720721855092 ) ) ;
#22966=CARTESIAN_POINT ( 'NONE',  ( 43.31606138205700063, 3.296535697557910538, 65.33616386252352015 ) ) ;
#23017=ORIENTED_EDGE ( 'NONE', *, *, #14150, .F. ) ;
#23023=LINE ( 'NONE', #19413, #15548 ) ;
#23030=ORIENTED_EDGE ( 'NONE', *, *, #1756, .F. ) ;
#23047=AXIS2_PLACEMENT_3D ( 'NONE', #1039, #22821, #17032 ) ;
#23055=CARTESIAN_POINT ( 'NONE',  ( 35.31606138205700773, 7.535758204303438568, 66.26723409915207696 ) ) ;
#23085=CARTESIAN_POINT ( 'NONE',  ( 33.31606138205700773, 3.392460599465057403, 64.84545171350526971 ) ) ;
#23092=MECHANICAL_DESIGN_GEOMETRIC_PRESENTATION_REPRESENTATION('',(#16512),#21048);
#23102=PLANE ( 'NONE',  #7187 ) ;
#23124=VERTEX_POINT ( 'NONE', #3793 ) ;
#23127=LINE ( 'NONE', #11811, #24553 ) ;
#23137=AXIS2_PLACEMENT_3D ( 'NONE', #1256, #16455, #20585 ) ;
#23165=ORIENTED_EDGE ( 'NONE', *, *, #22490, .T. ) ;
#23185=ORIENTED_EDGE ( 'NONE', *, *, #6762, .F. ) ;
#23215=PLANE ( 'NONE',  #21269 ) ;
#23226=DIRECTION ( 'NONE',  ( 0.000000000000000000, -0.1918498038142812112, 0.9814242980364923374 ) ) ;
#23265=EDGE_CURVE ( 'NONE', #1793, #16154, #4188, .T. ) ;
#23272=EDGE_LOOP ( 'NONE', ( #4065, #1919, #23417, #14545 ) ) ;
#23277=DIRECTION ( 'NONE',  ( 0.000000000000000000, 0.7540134720837716742, 0.6568589528324746407 ) ) ;
#23307=PRODUCT_DEFINITION ( 'UNKNOWN', '', #19938, #12130 ) ;
#23325=DIRECTION ( 'NONE',  ( 0.000000000000000000, -0.7540134720837718962, -0.6568589528324743076 ) ) ;
#23341=ORIENTED_EDGE ( 'NONE', *, *, #19314, .F. ) ;
#23360=VERTEX_POINT ( 'NONE', #23055 ) ;
#23363=ORIENTED_EDGE ( 'NONE', *, *, #19791, .T. ) ;
#23370=CARTESIAN_POINT ( 'NONE',  ( 33.31606138205700773, 10.06218483883314718, 67.80501292737497465 ) ) ;
#23373=VECTOR ( 'NONE', #3564, 1000.000000000000227 ) ;
#23375=ORIENTED_EDGE ( 'NONE', *, *, #12217, .T. ) ;
#23377=LINE ( 'NONE', #3801, #25386 ) ;
#23387=CARTESIAN_POINT ( 'NONE',  ( 41.31606138205700063, 14.21032488318011211, 61.14033482768515881 ) ) ;
#23403=EDGE_CURVE ( 'NONE', #18110, #16336, #22459, .T. ) ;
#23406=EDGE_CURVE ( 'NONE', #22767, #19154, #6495, .T. ) ;
#23412=ORIENTED_EDGE ( 'NONE', *, *, #4695, .F. ) ;
#23417=ORIENTED_EDGE ( 'NONE', *, *, #5849, .F. ) ;
#23422=EDGE_CURVE ( 'NONE', #19611, #13467, #12689, .T. ) ;
#23425=LINE ( 'NONE', #6044, #18874 ) ;
#23427=LINE ( 'NONE', #21502, #16848 ) ;
#23429=DIRECTION ( 'NONE',  ( 0.000000000000000000, -0.1918498038142821827, 0.9814242980364921154 ) ) ;
#23460=VECTOR ( 'NONE', #5773, 1000.000000000000227 ) ;
#23471=EDGE_LOOP ( 'NONE', ( #16424, #25274, #11902, #22834 ) ) ;
#23474=CARTESIAN_POINT ( 'NONE',  ( 35.31606138205700773, -20.93319939328399926, 43.78741072286599945 ) ) ;
#23479=ORIENTED_EDGE ( 'NONE', *, *, #15066, .F. ) ;
#23485=CYLINDRICAL_SURFACE ( 'NONE', #20076, 1.500000000000001332 ) ;
#23506=LINE ( 'NONE', #21328, #13083 ) ;
#23555=DIRECTION ( 'NONE',  ( 0.000000000000000000, 0.7540134720837717852, 0.6568589528324747517 ) ) ;
#23557=SURFACE_STYLE_FILL_AREA ( #3721 ) ;
#23582=DIRECTION ( 'NONE',  ( 0.000000000000000000, 0.7540134720837716742, 0.6568589528324746407 ) ) ;
#23617=LINE ( 'NONE', #21564, #8016 ) ;
#23654=ORIENTED_EDGE ( 'NONE', *, *, #3502, .F. ) ;
#23657=AXIS2_PLACEMENT_3D ( 'NONE', #15216, #13042, #7243 ) ;
#23673=ORIENTED_EDGE ( 'NONE', *, *, #24642, .F. ) ;
#23707=CARTESIAN_POINT ( 'NONE',  ( 35.31606138205700773, 2.715274261285174351, 65.05190033008260286 ) ) ;
#23745=ORIENTED_EDGE ( 'NONE', *, *, #14555, .T. ) ;
#23753=CARTESIAN_POINT ( 'NONE',  ( 33.31606138205700773, 1.535676793533870210, 63.36117568837578062 ) ) ;
#23776=CARTESIAN_POINT ( 'NONE',  ( 36.81606138205700063, -0.7263636227174442572, 61.39059882987834982 ) ) ;
#23778=ORIENTED_EDGE ( 'NONE', *, *, #22042, .F. ) ;
#23810=DIRECTION ( 'NONE',  ( 0.000000000000000000, 0.6568589528324746407, -0.7540134720837717852 ) ) ;
#23820=EDGE_CURVE ( 'NONE', #981, #14083, #22021, .T. ) ;
#23835=VECTOR ( 'NONE', #25270, 1000.000000000000227 ) ;
#23854=VERTEX_POINT ( 'NONE', #6681 ) ;
#23862=EDGE_CURVE ( 'NONE', #21235, #4126, #8377, .T. ) ;
#23863=VERTEX_POINT ( 'NONE', #10435 ) ;
#23873=ORIENTED_EDGE ( 'NONE', *, *, #18776, .F. ) ;
#23880=ORIENTED_EDGE ( 'NONE', *, *, #802, .T. ) ;
#23884=ORIENTED_EDGE ( 'NONE', *, *, #18105, .T. ) ;
#23886=EDGE_CURVE ( 'NONE', #24510, #8968, #7326, .T. ) ;
#23891=VERTEX_POINT ( 'NONE', #16727 ) ;
#23893=CARTESIAN_POINT ( 'NONE',  ( 33.31606138205700773, 3.099306811489555891, 65.29760936252343129 ) ) ;
#23948=ADVANCED_FACE ( 'NONE', ( #13132 ), #5145, .T. ) ;
#23950=DIRECTION ( 'NONE',  ( 0.000000000000000000, 0.6568589528324746407, -0.7540134720837717852 ) ) ;
#23954=VECTOR ( 'NONE', #24803, 1000.000000000000227 ) ;
#23962=PLANE ( 'NONE',  #19747 ) ;
#23963=AXIS2_PLACEMENT_3D ( 'NONE', #12975, #14286, #20211 ) ;
#23979=FACE_BOUND ( 'NONE', #2807, .T. ) ;
#23994=AXIS2_PLACEMENT_3D ( 'NONE', #171, #416, #5987 ) ;
#24006=EDGE_LOOP ( 'NONE', ( #19332, #19777, #25014, #18620 ) ) ;
#24008=CARTESIAN_POINT ( 'NONE',  ( 35.31606138205700773, 14.21032488318011211, 61.14033482768515881 ) ) ;
#24014=EDGE_LOOP ( 'NONE', ( #16677, #16030, #6236, #22031 ) ) ;
#24018=ORIENTED_EDGE ( 'NONE', *, *, #20550, .T. ) ;
#24050=LINE ( 'NONE', #14526, #12436 ) ;
#24053=ADVANCED_FACE ( 'NONE', ( #11202 ), #9526, .F. ) ;
#24069=EDGE_CURVE ( 'NONE', #18865, #20940, #13260, .T. ) ;
#24071=ORIENTED_EDGE ( 'NONE', *, *, #11134, .T. ) ;
#24076=DIRECTION ( 'NONE',  ( 0.000000000000000000, -0.6568589528324746407, 0.7540134720837716742 ) ) ;
#24097=ORIENTED_EDGE ( 'NONE', *, *, #22166, .T. ) ;
#24117=EDGE_CURVE ( 'NONE', #17790, #6859, #25068, .T. ) ;
#24134=DIRECTION ( 'NONE',  ( -1.000000000000000000, 0.000000000000000000, 0.000000000000000000 ) ) ;
#24147=VERTEX_POINT ( 'NONE', #11334 ) ;
#24174=CARTESIAN_POINT ( 'NONE',  ( 44.31606138205700063, 10.62769494289597993, 68.29765714199933768 ) ) ;
#24200=DIRECTION ( 'NONE',  ( 0.000000000000000000, 0.7540134720837725624, 0.6568589528324736415 ) ) ;
#24317=EDGE_CURVE ( 'NONE', #21235, #18110, #3707, .T. ) ;
#24325=VECTOR ( 'NONE', #2409, 1000.000000000000227 ) ;
#24340=VECTOR ( 'NONE', #15293, 1000.000000000000000 ) ;
#24343=VECTOR ( 'NONE', #4711, 1000.000000000000227 ) ;
#24405=EDGE_LOOP ( 'NONE', ( #17349, #16307, #7397, #3517 ) ) ;
#24413=DIRECTION ( 'NONE',  ( -1.000000000000000000, 0.000000000000000000, 0.000000000000000000 ) ) ;
#24428=LINE ( 'NONE', #5251, #2160 ) ;
#24432=CARTESIAN_POINT ( 'NONE',  ( 44.31606138205700063, -20.93319939328399926, 43.78741072286599945 ) ) ;
#24438=CARTESIAN_POINT ( 'NONE',  ( 33.31606138205700773, 3.043703737701412226, 64.67489359404071081 ) ) ;
#24445=EDGE_LOOP ( 'NONE', ( #21113, #9513, #4488, #22465, #10157, #19408, #21710, #13986, #1382, #2264, #21163, #11529, #239, #2222, #9997, #25338 ) ) ;
#24448=DIRECTION ( 'NONE',  ( 0.000000000000000000, 0.6568589528324745297, -0.7540134720837717852 ) ) ;
#24459=LINE ( 'NONE', #20619, #7639 ) ;
#24505=CARTESIAN_POINT ( 'NONE',  ( 35.31606138205700773, 7.535758204303438568, 66.26723409915207696 ) ) ;
#24506=DIRECTION ( 'NONE',  ( -1.000000000000000000, 0.000000000000000000, 0.000000000000000000 ) ) ;
#24510=VERTEX_POINT ( 'NONE', #12979 ) ;
#24552=CIRCLE ( 'NONE', #5655, 1.500000000000001332 ) ;
#24553=VECTOR ( 'NONE', #5499, 1000.000000000000227 ) ;
#24584=LINE ( 'NONE', #20369, #22785 ) ;
#24642=EDGE_CURVE ( 'NONE', #22382, #22220, #24913, .T. ) ;
#24648=ORIENTED_EDGE ( 'NONE', *, *, #7926, .T. ) ;
#24659=VECTOR ( 'NONE', #8283, 1000.000000000000227 ) ;
#24693=VERTEX_POINT ( 'NONE', #3797 ) ;
#24748=FACE_OUTER_BOUND ( 'NONE', #2084, .T. ) ;
#24774=EDGE_CURVE ( 'NONE', #12000, #9479, #7032, .T. ) ;
#24788=PLANE ( 'NONE',  #5060 ) ;
#24794=EDGE_LOOP ( 'NONE', ( #8839, #18050, #22797, #4503 ) ) ;
#24798=EDGE_CURVE ( 'NONE', #23124, #5934, #12062, .T. ) ;
#24800=ORIENTED_EDGE ( 'NONE', *, *, #11627, .F. ) ;
#24803=DIRECTION ( 'NONE',  ( 0.000000000000000000, -0.1918498038142812112, 0.9814242980364923374 ) ) ;
#24820=CARTESIAN_POINT ( 'NONE',  ( 43.31606138205700063, 7.283211578144648257, 66.04722806671131252 ) ) ;
#24830=ADVANCED_FACE ( 'NONE', ( #13854 ), #19909, .F. ) ;
#24836=PLANE ( 'NONE',  #17926 ) ;
#24848=CARTESIAN_POINT ( 'NONE',  ( 33.31606138205700773, 2.715274261285174351, 65.05190033008260286 ) ) ;
#24866=FACE_OUTER_BOUND ( 'NONE', #19269, .T. ) ;
#24885=ORIENTED_EDGE ( 'NONE', *, *, #11295, .T. ) ;
#24906=VERTEX_POINT ( 'NONE', #25177 ) ;
#24913=LINE ( 'NONE', #21589, #13622 ) ;
#24941=CARTESIAN_POINT ( 'NONE',  ( 43.31606138205700063, 3.296535697557910538, 65.33616386252352015 ) ) ;
#24949=EDGE_LOOP ( 'NONE', ( #13327, #9981, #15084, #12191 ) ) ;
#24953=CLOSED_SHELL ( 'NONE', ( #22300, #1504, #8768, #21537, #19546, #10080, #5384, #388, #11019, #18854, #24830, #21077, #13339, #16696, #16487, #4844, #2965, #6399, #3316, #9817, #15064, #15946, #4692, #23948, #7278, #3061, #866, #2667, #24053, #10225, #5766, #20137, #14176, #14156, #13835, #13274, #18375, #21547, #1117, #8252, #15294, #1453, #2488, #2289, #5960, #25413, #25015, #13455, #16823, #15992, #9449, #14116, #19169, #17858, #6914, #22303, #20427, #21076 ) ) ;
#25014=ORIENTED_EDGE ( 'NONE', *, *, #9198, .F. ) ;
#25015=ADVANCED_FACE ( 'NONE', ( #9379 ), #3307, .T. ) ;
#25027=ORIENTED_EDGE ( 'NONE', *, *, #1555, .F. ) ;
#25053=LINE ( 'NONE', #23387, #9159 ) ;
#25068=LINE ( 'NONE', #21355, #411 ) ;
#25109=ORIENTED_EDGE ( 'NONE', *, *, #649, .T. ) ;
#25115=SURFACE_STYLE_FILL_AREA ( #9699 ) ;
#25135=VERTEX_POINT ( 'NONE', #572 ) ;
#25150=AXIS2_PLACEMENT_3D ( 'NONE', #276, #10477, #21680 ) ;
#25157=DIRECTION ( 'NONE',  ( 0.000000000000000000, 0.7540134720837717852, 0.6568589528324746407 ) ) ;
#25175=CARTESIAN_POINT ( 'NONE',  ( 43.31606138205700063, 7.611641054560886133, 65.67022133066943468 ) ) ;
#25177=CARTESIAN_POINT ( 'NONE',  ( 41.31606138205700063, 3.296535697557906985, 65.33616386252352015 ) ) ;
#25196=CARTESIAN_POINT ( 'NONE',  ( 44.31606138205700063, -20.55619265724211076, 44.11584019928223910 ) ) ;
#25201=EDGE_LOOP ( 'NONE', ( #13923, #23412, #11583, #2747 ) ) ;
#25261=LINE ( 'NONE', #5329, #17654 ) ;
#25270=DIRECTION ( 'NONE',  ( 0.000000000000000000, -0.7540134720837717852, -0.6568589528324746407 ) ) ;
#25274=ORIENTED_EDGE ( 'NONE', *, *, #2795, .F. ) ;
#25289=CARTESIAN_POINT ( 'NONE',  ( 32.31606138205700063, 10.62769494289597993, 68.29765714199933768 ) ) ;
#25296=DIRECTION ( 'NONE',  ( 0.000000000000000000, 0.7540134720837725624, 0.6568589528324736415 ) ) ;
#25300=ORIENTED_EDGE ( 'NONE', *, *, #25471, .F. ) ;
#25331=ORIENTED_EDGE ( 'NONE', *, *, #1555, .T. ) ;
#25338=ORIENTED_EDGE ( 'NONE', *, *, #19689, .T. ) ;
#25355=CARTESIAN_POINT ( 'NONE',  ( 44.31606138205700063, 10.29926546647973851, 68.67466387804121553 ) ) ;
#25362=EDGE_LOOP ( 'NONE', ( #19835, #17732, #20309, #21463 ) ) ;
#25367=AXIS2_PLACEMENT_3D ( 'NONE', #5319, #9574, #23325 ) ;
#25373=CARTESIAN_POINT ( 'NONE',  ( 43.31606138205700063, 7.282926244446933595, 65.60596383066929604 ) ) ;
#25386=VECTOR ( 'NONE', #19527, 1000.000000000000227 ) ;
#25387=CYLINDRICAL_SURFACE ( 'NONE', #25465, 1.500000000000001332 ) ;
#25389=FACE_OUTER_BOUND ( 'NONE', #7229, .T. ) ;
#25391=ORIENTED_EDGE ( 'NONE', *, *, #19638, .T. ) ;
#25403=AXIS2_PLACEMENT_3D ( 'NONE', #22030, #17928, #24076 ) ;
#25408=DIRECTION ( 'NONE',  ( 1.000000000000000000, 0.000000000000000000, 0.000000000000000000 ) ) ;
#25413=ADVANCED_FACE ( 'NONE', ( #9722 ), #16346, .T. ) ;
#25427=AXIS2_PLACEMENT_3D ( 'NONE', #16204, #15949, #6303 ) ;
#25436=LINE ( 'NONE', #67, #10404 ) ;
#25454=DIRECTION ( 'NONE',  ( 0.000000000000000000, 0.7540134720837717852, 0.6568589528324746407 ) ) ;
#25465=AXIS2_PLACEMENT_3D ( 'NONE', #8028, #1947, #21799 ) ;
#25471=EDGE_CURVE ( 'NONE', #18988, #22382, #5703, .T. ) ;
#25472=EDGE_LOOP ( 'NONE', ( #11793, #11364 ) ) ;
ENDSEC;
END-ISO-10303-21;
